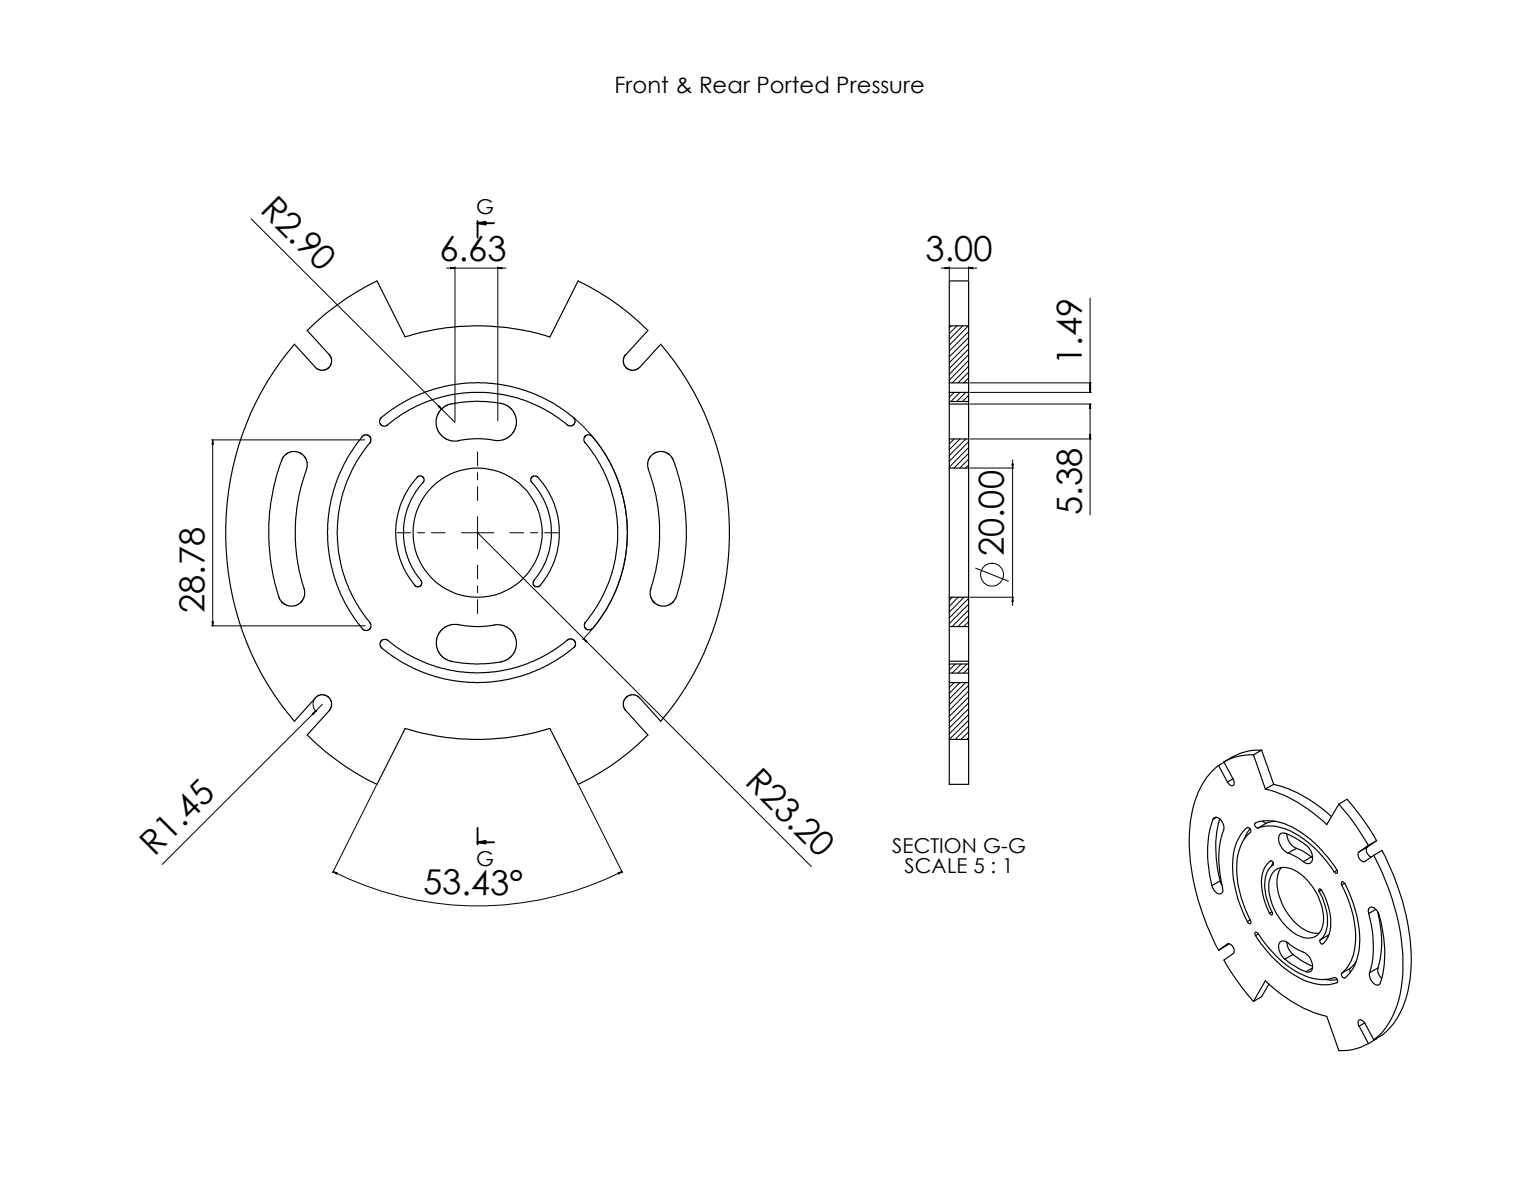
ISO-10303-21;
HEADER;
FILE_DESCRIPTION (('STEP AP214'),
    '1' );
FILE_NAME ('Front & Rear Ported Pressure.step',
    '2026-10-18T20:16:25',
    ( '' ),
    ( '' ),
    'SwSTEP 2.0',
    'SolidWorks 2025',
    '' );
FILE_SCHEMA (( 'AUTOMOTIVE_DESIGN' ));
ENDSEC;

DATA;
#15=ORIENTED_EDGE ( 'NONE', *, *, #5581, .T. ) ;
#25=AXIS2_PLACEMENT_3D ( 'NONE', #902, #17278, #15225 ) ;
#26=CARTESIAN_POINT ( 'NONE',  ( 30.75232512042845556, -9.966982604840845639, 1.500000000000000000 ) ) ;
#30=EDGE_CURVE ( 'NONE', #13253, #5262, #636, .T. ) ;
#59=ORIENTED_EDGE ( 'NONE', *, *, #6132, .F. ) ;
#63=EDGE_CURVE ( 'NONE', #25705, #14162, #9332, .T. ) ;
#81=CARTESIAN_POINT ( 'NONE',  ( -1.073881485057447405, -0.9711784013058452070, 1.500000000000000000 ) ) ;
#121=VECTOR ( 'NONE', #17231, 1000.000000000000000 ) ;
#142=AXIS2_PLACEMENT_3D ( 'NONE', #29835, #3468, #10482 ) ;
#156=DIRECTION ( 'NONE',  ( -0.000000000000000000, 0.000000000000000000, 1.000000000000000000 ) ) ;
#172=ORIENTED_EDGE ( 'NONE', *, *, #2713, .T. ) ;
#180=DIRECTION ( 'NONE',  ( 1.000000000000000000, 0.000000000000000000, 0.000000000000000000 ) ) ;
#190=DIRECTION ( 'NONE',  ( -0.6707505147970024284, 0.7416830501633134842, 0.000000000000000000 ) ) ;
#192=EDGE_CURVE ( 'NONE', #26671, #20986, #30262, .T. ) ;
#204=ORIENTED_EDGE ( 'NONE', *, *, #13604, .T. ) ;
#206=CIRCLE ( 'NONE', #4196, 0.7441270634457181066 ) ;
#213=CARTESIAN_POINT ( 'NONE',  ( -19.54426622602688113, -37.07991288358296345, -1.499999999999999778 ) ) ;
#244=CIRCLE ( 'NONE', #26653, 0.7441270634457198829 ) ;
#248=ORIENTED_EDGE ( 'NONE', *, *, #13418, .T. ) ;
#251=EDGE_CURVE ( 'NONE', #24781, #12321, #29562, .T. ) ;
#252=LINE ( 'NONE', #7437, #4085 ) ;
#265=EDGE_CURVE ( 'NONE', #30031, #12516, #9139, .T. ) ;
#274=DIRECTION ( 'NONE',  ( -0.000000000000000000, 0.000000000000000000, 1.000000000000000000 ) ) ;
#282=DIRECTION ( 'NONE',  ( -0.000000000000000000, -0.000000000000000000, -1.000000000000000000 ) ) ;
#288=AXIS2_PLACEMENT_3D ( 'NONE', #22323, #7993, #29353 ) ;
#292=ORIENTED_EDGE ( 'NONE', *, *, #27712, .F. ) ;
#317=AXIS2_PLACEMENT_3D ( 'NONE', #8530, #7913, #10548 ) ;
#320=DIRECTION ( 'NONE',  ( -1.000000000000000000, 0.000000000000000000, 0.000000000000000000 ) ) ;
#322=CYLINDRICAL_SURFACE ( 'NONE', #25724, 20.32284676574538906 ) ;
#374=CIRCLE ( 'NONE', #21296, 0.7441270634457181066 ) ;
#388=FACE_OUTER_BOUND ( 'NONE', #26241, .T. ) ;
#408=DIRECTION ( 'NONE',  ( -1.000000000000000000, 0.000000000000000000, 0.000000000000000000 ) ) ;
#409=ORIENTED_EDGE ( 'NONE', *, *, #20131, .F. ) ;
#423=AXIS2_PLACEMENT_3D ( 'NONE', #5251, #14749, #10546 ) ;
#429=EDGE_CURVE ( 'NONE', #25490, #7103, #10636, .T. ) ;
#442=ORIENTED_EDGE ( 'NONE', *, *, #12082, .T. ) ;
#450=EDGE_CURVE ( 'NONE', #9427, #25685, #22270, .T. ) ;
#468=CYLINDRICAL_SURFACE ( 'NONE', #18787, 2.898871837527149165 ) ;
#479=VERTEX_POINT ( 'NONE', #10583 ) ;
#481=CYLINDRICAL_SURFACE ( 'NONE', #1478, 0.6002263538043648428 ) ;
#486=ORIENTED_EDGE ( 'NONE', *, *, #11751, .F. ) ;
#491=LINE ( 'NONE', #29032, #2354 ) ;
#494=FACE_OUTER_BOUND ( 'NONE', #15914, .T. ) ;
#512=ORIENTED_EDGE ( 'NONE', *, *, #14149, .F. ) ;
#514=CARTESIAN_POINT ( 'NONE',  ( 9.216505592218814158, -7.781333699927420966, -1.500000000000000000 ) ) ;
#517=ORIENTED_EDGE ( 'NONE', *, *, #25356, .F. ) ;
#518=FACE_OUTER_BOUND ( 'NONE', #7310, .T. ) ;
#558=LINE ( 'NONE', #12121, #27803 ) ;
#568=LINE ( 'NONE', #26949, #28027 ) ;
#570=ORIENTED_EDGE ( 'NONE', *, *, #6962, .T. ) ;
#574=ADVANCED_BREP_SHAPE_REPRESENTATION ( '', ( #2768, #7396 ), #910 ) ;
#584=VERTEX_POINT ( 'NONE', #5059 ) ;
#597=ADVANCED_FACE ( 'NONE', ( #17058 ), #18881, .F. ) ;
#613=CARTESIAN_POINT ( 'NONE',  ( -4.100931858250860707, -19.90478481566557534, 1.500000000000000000 ) ) ;
#629=ORIENTED_EDGE ( 'NONE', *, *, #8754, .F. ) ;
#636=LINE ( 'NONE', #3142, #22778 ) ;
#652=EDGE_CURVE ( 'NONE', #15421, #2309, #4171, .T. ) ;
#663=CARTESIAN_POINT ( 'NONE',  ( -43.34097750826428097, -11.89502811014147987, -1.500000000000000444 ) ) ;
#666=CARTESIAN_POINT ( 'NONE',  ( -17.26937953831790651, 14.36006998371489551, -1.500000000000000000 ) ) ;
#686=FACE_OUTER_BOUND ( 'NONE', #13708, .T. ) ;
#701=CARTESIAN_POINT ( 'NONE',  ( -1.073881485057738949, 0.9711784013061123266, -1.500000000000000000 ) ) ;
#703=CARTESIAN_POINT ( 'NONE',  ( 26.36764545593177544, -31.31467416275353344, -1.500000000000000000 ) ) ;
#706=CARTESIAN_POINT ( 'NONE',  ( 24.03057240117691862, -26.57182937991349903, 1.500000000000000000 ) ) ;
#708=DIRECTION ( 'NONE',  ( 1.000000000000000000, 0.000000000000000000, 0.000000000000000000 ) ) ;
#717=DIRECTION ( 'NONE',  ( -0.000000000000000000, -0.000000000000000000, -1.000000000000000000 ) ) ;
#722=EDGE_LOOP ( 'NONE', ( #5355, #17765, #14254, #19084 ) ) ;
#733=( BOUNDED_CURVE ( )  B_SPLINE_CURVE ( 3, ( #29605, #26969, #8239, #8560 ),
 .UNSPECIFIED., .F., .T. ) 
 B_SPLINE_CURVE_WITH_KNOTS ( ( 4, 4 ),
 ( 3.955359442064654285, 5.469418518704724619 ),
 .UNSPECIFIED. ) 
 CURVE ( )  GEOMETRIC_REPRESENTATION_ITEM ( )  RATIONAL_B_SPLINE_CURVE ( ( 1.000000000000000000, 0.8179194830933629312, 0.8179194830933629312, 1.000000000000000000 ) ) 
 REPRESENTATION_ITEM ( '' )  );
#734=ORIENTED_EDGE ( 'NONE', *, *, #10715, .F. ) ;
#751=ADVANCED_FACE ( 'NONE', ( #22199 ), #1146, .F. ) ;
#763=ORIENTED_EDGE ( 'NONE', *, *, #27893, .T. ) ;
#775=CARTESIAN_POINT ( 'NONE',  ( 13.93942108199810193, -16.65122935894600076, 1.500000000000000000 ) ) ;
#791=ADVANCED_FACE ( 'NONE', ( #25481 ), #27968, .F. ) ;
#793=CIRCLE ( 'NONE', #3294, 2.061368542273053883 ) ;
#800=FACE_OUTER_BOUND ( 'NONE', #27813, .T. ) ;
#801=CARTESIAN_POINT ( 'NONE',  ( -4.163336342344337027E-14, -1.387778780781445676E-14, 1.500000000000000000 ) ) ;
#821=CARTESIAN_POINT ( 'NONE',  ( 0.000000000000000000, 0.000000000000000000, -1.500000000000000000 ) ) ;
#848=ORIENTED_EDGE ( 'NONE', *, *, #26955, .T. ) ;
#855=CIRCLE ( 'NONE', #18782, 1.447898107987198646 ) ;
#864=DIRECTION ( 'NONE',  ( -1.000000000000000000, 0.000000000000000000, 0.000000000000000000 ) ) ;
#871=AXIS2_PLACEMENT_3D ( 'NONE', #23570, #30756, #18919 ) ;
#876=CARTESIAN_POINT ( 'NONE',  ( 8.419710366748642372, 7.777014463793876509, 1.500000000000000000 ) ) ;
#889=VECTOR ( 'NONE', #15046, 1000.000000000000000 ) ;
#902=CARTESIAN_POINT ( 'NONE',  ( -4.163336342344337027E-14, -1.387778780781445676E-14, 1.500000000000000000 ) ) ;
#907=EDGE_CURVE ( 'NONE', #20436, #24781, #5018, .T. ) ;
#910=( GEOMETRIC_REPRESENTATION_CONTEXT ( 3 ) GLOBAL_UNCERTAINTY_ASSIGNED_CONTEXT ( ( #13624 ) ) GLOBAL_UNIT_ASSIGNED_CONTEXT ( ( #14769, #3081, #22254 ) ) REPRESENTATION_CONTEXT ( 'NONE', 'WORKASPACE' ) );
#927=ORIENTED_EDGE ( 'NONE', *, *, #27710, .F. ) ;
#953=EDGE_CURVE ( 'NONE', #29550, #14341, #3391, .T. ) ;
#955=CARTESIAN_POINT ( 'NONE',  ( -4.163336342344337027E-14, -1.387778780781445676E-14, -1.500000000000000000 ) ) ;
#958=CARTESIAN_POINT ( 'NONE',  ( -15.57266529552203416, -38.96488032230103471, 1.500000000000000000 ) ) ;
#973=CARTESIAN_POINT ( 'NONE',  ( -17.26937953831790651, 14.36006998371489551, 1.500000000000000000 ) ) ;
#986=CARTESIAN_POINT ( 'NONE',  ( -11.46182693247433804, -1.387778780781445676E-14, 1.500000000000000000 ) ) ;
#993=AXIS2_PLACEMENT_3D ( 'NONE', #30844, #28672, #23658 ) ;
#994=CARTESIAN_POINT ( 'NONE',  ( -23.17581250239728519, -34.50630206824673252, 1.499999999999999778 ) ) ;
#1017=AXIS2_PLACEMENT_3D ( 'NONE', #1740, #20609, #28248 ) ;
#1028=CYLINDRICAL_SURFACE ( 'NONE', #9384, 0.7441270634457198829 ) ;
#1036=EDGE_CURVE ( 'NONE', #3590, #15421, #14834, .T. ) ;
#1037=DIRECTION ( 'NONE',  ( -1.000000000000000000, 0.000000000000000000, 0.000000000000000000 ) ) ;
#1041=CARTESIAN_POINT ( 'NONE',  ( -43.34097750826428097, -11.89502811014148342, -1.500000000000000444 ) ) ;
#1046=DIRECTION ( 'NONE',  ( -0.000000000000000000, -0.000000000000000000, -1.000000000000000000 ) ) ;
#1049=ORIENTED_EDGE ( 'NONE', *, *, #3733, .T. ) ;
#1059=ORIENTED_EDGE ( 'NONE', *, *, #26955, .F. ) ;
#1073=CARTESIAN_POINT ( 'NONE',  ( -28.79137815760242702, -9.331429872129930914, 1.500000000000000000 ) ) ;
#1076=FACE_BOUND ( 'NONE', #3866, .T. ) ;
#1078=CARTESIAN_POINT ( 'NONE',  ( 15.57266529552203416, -38.96488032230103471, -1.500000000000000000 ) ) ;
#1105=VERTEX_POINT ( 'NONE', #15603 ) ;
#1106=DIRECTION ( 'NONE',  ( -1.000000000000000000, 0.000000000000000000, 0.000000000000000000 ) ) ;
#1108=DIRECTION ( 'NONE',  ( 1.000000000000000000, 0.000000000000000000, 0.000000000000000000 ) ) ;
#1113=AXIS2_PLACEMENT_3D ( 'NONE', #20021, #3967, #25158 ) ;
#1122=DIRECTION ( 'NONE',  ( 1.000000000000000000, 0.000000000000000000, 0.000000000000000000 ) ) ;
#1123=CARTESIAN_POINT ( 'NONE',  ( 24.03057240117691862, -26.57182937991349903, -1.500000000000000000 ) ) ;
#1135=VECTOR ( 'NONE', #24120, 1000.000000000000000 ) ;
#1138=CARTESIAN_POINT ( 'NONE',  ( -24.03057240117691862, -26.57182937991349903, 1.500000000000000000 ) ) ;
#1146=CYLINDRICAL_SURFACE ( 'NONE', #13138, 0.7441270634457181066 ) ;
#1158=ORIENTED_EDGE ( 'NONE', *, *, #15067, .F. ) ;
#1167=ORIENTED_EDGE ( 'NONE', *, *, #6161, .F. ) ;
#1172=EDGE_CURVE ( 'NONE', #27927, #23361, #4939, .T. ) ;
#1176=AXIS2_PLACEMENT_3D ( 'NONE', #4448, #24929, #1953 ) ;
#1177=ADVANCED_FACE ( 'NONE', ( #4517, #28690, #28535, #7328, #20890, #16837, #14027, #23530, #16679, #2176, #11399, #13884 ), #7011, .F. ) ;
#1185=LINE ( 'NONE', #5548, #28491 ) ;
#1202=FACE_OUTER_BOUND ( 'NONE', #13290, .T. ) ;
#1205=ORIENTED_EDGE ( 'NONE', *, *, #1997, .F. ) ;
#1212=DIRECTION ( 'NONE',  ( 1.000000000000000000, 0.000000000000000000, 0.000000000000000000 ) ) ;
#1236=FACE_OUTER_BOUND ( 'NONE', #7384, .T. ) ;
#1264=EDGE_CURVE ( 'NONE', #6747, #8400, #30302, .T. ) ;
#1265=LINE ( 'NONE', #18424, #21036 ) ;
#1272=DIRECTION ( 'NONE',  ( -0.000000000000000000, 0.000000000000000000, 1.000000000000000000 ) ) ;
#1275=CARTESIAN_POINT ( 'NONE',  ( -4.163336342344337027E-14, -1.387778780781445676E-14, 1.500000000000000000 ) ) ;
#1276=ORIENTED_EDGE ( 'NONE', *, *, #27924, .F. ) ;
#1277=ORIENTED_EDGE ( 'NONE', *, *, #5949, .F. ) ;
#1284=DIRECTION ( 'NONE',  ( -1.000000000000000000, 0.000000000000000000, 0.000000000000000000 ) ) ;
#1304=ORIENTED_EDGE ( 'NONE', *, *, #26374, .T. ) ;
#1329=DIRECTION ( 'NONE',  ( -1.000000000000000000, 0.000000000000000000, 0.000000000000000000 ) ) ;
#1341=CARTESIAN_POINT ( 'NONE',  ( -22.95669091611927826, -27.54300778121952220, 1.500000000000000000 ) ) ;
#1346=AXIS2_PLACEMENT_3D ( 'NONE', #18219, #6660, #16178 ) ;
#1352=VERTEX_POINT ( 'NONE', #5606 ) ;
#1358=DIRECTION ( 'NONE',  ( 1.000000000000000000, 0.000000000000000000, 0.000000000000000000 ) ) ;
#1360=ORIENTED_EDGE ( 'NONE', *, *, #7124, .F. ) ;
#1383=ADVANCED_FACE ( 'NONE', ( #20409, #22433, #24933, #13410, #30077, #1076, #24770, #15720, #11202, #3569, #10909, #15409 ), #29618, .T. ) ;
#1394=AXIS2_PLACEMENT_3D ( 'NONE', #19673, #26872, #10321 ) ;
#1397=CARTESIAN_POINT ( 'NONE',  ( 8.860628911697515875, 8.184276679720483116, 1.500000000000000000 ) ) ;
#1411=ORIENTED_EDGE ( 'NONE', *, *, #14365, .T. ) ;
#1416=LINE ( 'NONE', #3591, #23261 ) ;
#1427=CYLINDRICAL_SURFACE ( 'NONE', #14286, 0.7441270634457319844 ) ;
#1428=DIRECTION ( 'NONE',  ( -0.000000000000000000, -0.000000000000000000, -1.000000000000000000 ) ) ;
#1443=( LENGTH_UNIT ( ) NAMED_UNIT ( * ) SI_UNIT ( .MILLI., .METRE. ) );
#1449=ADVANCED_FACE ( 'NONE', ( #1236 ), #15568, .F. ) ;
#1460=CIRCLE ( 'NONE', #27926, 0.7441270634456903510 ) ;
#1462=ORIENTED_EDGE ( 'NONE', *, *, #19357, .F. ) ;
#1469=DIRECTION ( 'NONE',  ( -1.000000000000000000, 0.000000000000000000, 0.000000000000000000 ) ) ;
#1473=CIRCLE ( 'NONE', #23359, 2.061368542273053883 ) ;
#1478=AXIS2_PLACEMENT_3D ( 'NONE', #12501, #7807, #4847 ) ;
#1490=LINE ( 'NONE', #21948, #12448 ) ;
#1499=LINE ( 'NONE', #27688, #26304 ) ;
#1505=LINE ( 'NONE', #11014, #27746 ) ;
#1510=CARTESIAN_POINT ( 'NONE',  ( -16.69721919944057831, 13.88429941593312122, 1.500000000000000000 ) ) ;
#1513=VERTEX_POINT ( 'NONE', #16184 ) ;
#1514=ORIENTED_EDGE ( 'NONE', *, *, #15762, .F. ) ;
#1519=DIRECTION ( 'NONE',  ( -0.000000000000000000, 0.000000000000000000, 1.000000000000000000 ) ) ;
#1523=EDGE_LOOP ( 'NONE', ( #7018, #9466, #4233, #11567 ) ) ;
#1537=CARTESIAN_POINT ( 'NONE',  ( -11.21147646446735102, 30.29926891764210595, 1.500000000000000000 ) ) ;
#1542=DIRECTION ( 'NONE',  ( -0.000000000000000000, -0.000000000000000000, -1.000000000000000000 ) ) ;
#1571=ORIENTED_EDGE ( 'NONE', *, *, #2711, .T. ) ;
#1582=ORIENTED_EDGE ( 'NONE', *, *, #3226, .T. ) ;
#1596=DIRECTION ( 'NONE',  ( -0.000000000000000000, 0.000000000000000000, 1.000000000000000000 ) ) ;
#1611=EDGE_LOOP ( 'NONE', ( #27625, #4985, #27472, #29846 ) ) ;
#1625=DIRECTION ( 'NONE',  ( 1.000000000000000000, 0.000000000000000000, 0.000000000000000000 ) ) ;
#1632=DIRECTION ( 'NONE',  ( 1.000000000000000000, 0.000000000000000000, 0.000000000000000000 ) ) ;
#1633=VECTOR ( 'NONE', #3197, 1000.000000000000000 ) ;
#1651=DIRECTION ( 'NONE',  ( -0.000000000000000000, -0.000000000000000000, -1.000000000000000000 ) ) ;
#1675=FACE_OUTER_BOUND ( 'NONE', #11524, .T. ) ;
#1682=CARTESIAN_POINT ( 'NONE',  ( 17.79239818699415920, 14.89473990422378158, 1.500000000000000000 ) ) ;
#1707=CARTESIAN_POINT ( 'NONE',  ( -4.163336342344337027E-14, -1.387778780781445676E-14, -1.500000000000000000 ) ) ;
#1719=ORIENTED_EDGE ( 'NONE', *, *, #13952, .T. ) ;
#1725=VERTEX_POINT ( 'NONE', #12127 ) ;
#1727=CIRCLE ( 'NONE', #29633, 23.20393738267273420 ) ;
#1740=CARTESIAN_POINT ( 'NONE',  ( -4.163336342344337027E-14, 1.387778780781445676E-14, -1.500000000000000000 ) ) ;
#1743=ORIENTED_EDGE ( 'NONE', *, *, #12996, .F. ) ;
#1761=ADVANCED_FACE ( 'NONE', ( #19447 ), #14758, .F. ) ;
#1782=DIRECTION ( 'NONE',  ( -0.000000000000000000, -0.000000000000000000, -1.000000000000000000 ) ) ;
#1788=CARTESIAN_POINT ( 'NONE',  ( 17.84153987719590972, -14.83584055149750114, 1.500000000000000000 ) ) ;
#1800=CARTESIAN_POINT ( 'NONE',  ( 3.637110358602582583, 19.99473753024312117, 1.500000000000000000 ) ) ;
#1809=AXIS2_PLACEMENT_3D ( 'NONE', #13199, #12740, #10549 ) ;
#1821=CIRCLE ( 'NONE', #9786, 0.7441270634457337607 ) ;
#1831=CARTESIAN_POINT ( 'NONE',  ( 11.21147646446735102, 30.29926891764210595, -1.500000000000000000 ) ) ;
#1833=ORIENTED_EDGE ( 'NONE', *, *, #13418, .F. ) ;
#1834=AXIS2_PLACEMENT_3D ( 'NONE', #801, #3775, #24978 ) ;
#1851=CARTESIAN_POINT ( 'NONE',  ( -25.10445388623454477, 25.60065097860747585, -1.500000000000000000 ) ) ;
#1854=CARTESIAN_POINT ( 'NONE',  ( -23.20393738267338790, 0.000000000000000000, 1.500000000000000000 ) ) ;
#1856=ORIENTED_EDGE ( 'NONE', *, *, #17785, .F. ) ;
#1862=VECTOR ( 'NONE', #12585, 1000.000000000000000 ) ;
#1871=AXIS2_PLACEMENT_3D ( 'NONE', #12190, #16553, #28887 ) ;
#1876=ORIENTED_EDGE ( 'NONE', *, *, #23476, .F. ) ;
#1879=CIRCLE ( 'NONE', #15838, 1.447898107987198646 ) ;
#1884=VECTOR ( 'NONE', #29889, 1000.000000000000000 ) ;
#1914=CARTESIAN_POINT ( 'NONE',  ( -28.79137815760242702, -9.331429872129930914, 1.500000000000000000 ) ) ;
#1917=CARTESIAN_POINT ( 'NONE',  ( -25.10445388623454477, -25.60065097860747585, 1.500000000000000000 ) ) ;
#1921=AXIS2_PLACEMENT_3D ( 'NONE', #25373, #30355, #8997 ) ;
#1938=VECTOR ( 'NONE', #25198, 1000.000000000000000 ) ;
#1945=PLANE ( 'NONE',  #16481 ) ;
#1946=DIRECTION ( 'NONE',  ( 1.000000000000000000, 0.000000000000000000, 0.000000000000000000 ) ) ;
#1951=DIRECTION ( 'NONE',  ( 1.000000000000000000, 0.000000000000000000, 0.000000000000000000 ) ) ;
#1953=DIRECTION ( 'NONE',  ( 1.000000000000000000, -5.780230957810361426E-15, 0.000000000000000000 ) ) ;
#1997=EDGE_CURVE ( 'NONE', #27352, #27365, #19892, .T. ) ;
#2002=CARTESIAN_POINT ( 'NONE',  ( -13.88429941593315853, -16.69721919944146649, 1.500000000000000000 ) ) ;
#2003=ORIENTED_EDGE ( 'NONE', *, *, #16264, .T. ) ;
#2015=DIRECTION ( 'NONE',  ( -0.000000000000000000, -0.000000000000000000, -1.000000000000000000 ) ) ;
#2017=ORIENTED_EDGE ( 'NONE', *, *, #10988, .T. ) ;
#2042=ORIENTED_EDGE ( 'NONE', *, *, #21748, .F. ) ;
#2079=CARTESIAN_POINT ( 'NONE',  ( 28.79137815760242702, -9.331429872129930914, -1.500000000000000000 ) ) ;
#2090=DIRECTION ( 'NONE',  ( 1.000000000000000000, 0.000000000000000000, 0.000000000000000000 ) ) ;
#2108=CARTESIAN_POINT ( 'NONE',  ( -10.00000000000004263, 1.387778780781445676E-14, 1.500000000000000000 ) ) ;
#2110=EDGE_CURVE ( 'NONE', #16733, #28141, #22382, .T. ) ;
#2111=DIRECTION ( 'NONE',  ( 1.000000000000000000, 0.000000000000000000, 0.000000000000000000 ) ) ;
#2117=EDGE_CURVE ( 'NONE', #28435, #9405, #12931, .T. ) ;
#2125=VECTOR ( 'NONE', #190, 1000.000000000000000 ) ;
#2153=CIRCLE ( 'NONE', #29051, 37.60050224823048381 ) ;
#2171=VECTOR ( 'NONE', #29665, 1000.000000000000000 ) ;
#2176=FACE_BOUND ( 'NONE', #19630, .T. ) ;
#2206=CARTESIAN_POINT ( 'NONE',  ( 0.000000000000000000, 0.000000000000000000, 1.500000000000000000 ) ) ;
#2234=DIRECTION ( 'NONE',  ( 1.000000000000000000, 0.000000000000000000, 0.000000000000000000 ) ) ;
#2235=EDGE_CURVE ( 'NONE', #24520, #11332, #7958, .T. ) ;
#2255=ORIENTED_EDGE ( 'NONE', *, *, #24890, .F. ) ;
#2278=DIRECTION ( 'NONE',  ( -0.000000000000000000, -0.000000000000000000, -1.000000000000000000 ) ) ;
#2291=CARTESIAN_POINT ( 'NONE',  ( -22.95669091611927826, 27.54300778121952220, 1.500000000000000000 ) ) ;
#2309=VERTEX_POINT ( 'NONE', #18964 ) ;
#2354=VECTOR ( 'NONE', #3453, 1000.000000000000000 ) ;
#2370=CARTESIAN_POINT ( 'NONE',  ( 15.57266529552203416, 38.96488032230103471, -1.500000000000000000 ) ) ;
#2377=DIRECTION ( 'NONE',  ( -0.000000000000000000, -0.000000000000000000, -1.000000000000000000 ) ) ;
#2385=DIRECTION ( 'NONE',  ( -0.000000000000000000, -0.000000000000000000, -1.000000000000000000 ) ) ;
#2412=CARTESIAN_POINT ( 'NONE',  ( 15.57266529552201995, -38.96488032230103471, -1.500000000000000000 ) ) ;
#2414=AXIS2_PLACEMENT_3D ( 'NONE', #24888, #24716, #22392 ) ;
#2422=CARTESIAN_POINT ( 'NONE',  ( 17.79239818699415920, 14.89473990422378158, -1.500000000000000000 ) ) ;
#2423=ADVANCED_FACE ( 'NONE', ( #686 ), #28623, .T. ) ;
#2436=VECTOR ( 'NONE', #10712, 1000.000000000000000 ) ;
#2441=AXIS2_PLACEMENT_3D ( 'NONE', #28161, #6956, #2111 ) ;
#2447=LINE ( 'NONE', #11967, #11055 ) ;
#2453=CARTESIAN_POINT ( 'NONE',  ( 8.616279238414451314, -7.781333699927420966, 1.500000000000000000 ) ) ;
#2456=DIRECTION ( 'NONE',  ( -0.8932538319083086487, -0.4495526574063634095, 0.000000000000000000 ) ) ;
#2467=CARTESIAN_POINT ( 'NONE',  ( -22.95669091611927826, 27.54300778121952220, -1.500000000000000000 ) ) ;
#2480=AXIS2_PLACEMENT_3D ( 'NONE', #23136, #11458, #20941 ) ;
#2515=EDGE_CURVE ( 'NONE', #24825, #14826, #23426, .T. ) ;
#2517=VERTEX_POINT ( 'NONE', #21699 ) ;
#2528=DIRECTION ( 'NONE',  ( -0.000000000000000000, -0.000000000000000000, -1.000000000000000000 ) ) ;
#2536=CARTESIAN_POINT ( 'NONE',  ( -3.221450758838616757, 1.621276839356792454, -1.500000000000000000 ) ) ;
#2551=VERTEX_POINT ( 'NONE', #11908 ) ;
#2554=EDGE_LOOP ( 'NONE', ( #25894, #27667, #22850, #11057, #23980, #17264 ) ) ;
#2567=CARTESIAN_POINT ( 'NONE',  ( -26.36764545593177544, -31.31467416275353344, -1.500000000000000000 ) ) ;
#2584=DIRECTION ( 'NONE',  ( -1.000000000000000000, 0.000000000000000000, 0.000000000000000000 ) ) ;
#2593=VECTOR ( 'NONE', #21769, 1000.000000000000000 ) ;
#2601=CARTESIAN_POINT ( 'NONE',  ( -1.073881485057887497, 0.9711784013062738641, 1.500000000000000000 ) ) ;
#2604=LINE ( 'NONE', #2761, #2830 ) ;
#2618=CARTESIAN_POINT ( 'NONE',  ( 17.22181377297005866, 14.41708049311048789, -1.500000000000000000 ) ) ;
#2655=VECTOR ( 'NONE', #25234, 1000.000000000000000 ) ;
#2656=DIRECTION ( 'NONE',  ( -1.000000000000000000, 0.000000000000000000, 0.000000000000000000 ) ) ;
#2668=ORIENTED_EDGE ( 'NONE', *, *, #18963, .F. ) ;
#2672=ORIENTED_EDGE ( 'NONE', *, *, #5239, .T. ) ;
#2697=DIRECTION ( 'NONE',  ( -0.000000000000000000, 0.000000000000000000, 1.000000000000000000 ) ) ;
#2704=ORIENTED_EDGE ( 'NONE', *, *, #23249, .T. ) ;
#2710=CIRCLE ( 'NONE', #10186, 2.061368542273053883 ) ;
#2711=EDGE_CURVE ( 'NONE', #23725, #7065, #19746, .T. ) ;
#2713=EDGE_CURVE ( 'NONE', #26988, #12630, #8473, .T. ) ;
#2724=EDGE_CURVE ( 'NONE', #2309, #20990, #15232, .T. ) ;
#2755=LINE ( 'NONE', #12267, #2593 ) ;
#2761=CARTESIAN_POINT ( 'NONE',  ( 26.31795596221988376, 10.51822134874671022, 1.500000000000000000 ) ) ;
#2768=MANIFOLD_SOLID_BREP ( 'Boss-Extrude1', #19793 ) ;
#2773=CARTESIAN_POINT ( 'NONE',  ( -4.163336342344337027E-14, -1.387778780781445676E-14, 1.500000000000000000 ) ) ;
#2791=CARTESIAN_POINT ( 'NONE',  ( -19.54426622602688468, 37.07991288358297055, 1.499999999999999778 ) ) ;
#2795=DIRECTION ( 'NONE',  ( 1.000000000000000000, 0.000000000000000000, 0.000000000000000000 ) ) ;
#2826=FACE_OUTER_BOUND ( 'NONE', #17698, .T. ) ;
#2830=VECTOR ( 'NONE', #4942, 1000.000000000000000 ) ;
#2841=AXIS2_PLACEMENT_3D ( 'NONE', #29655, #26695, #8292 ) ;
#2843=CARTESIAN_POINT ( 'NONE',  ( -1.073881485057738949, -0.9711784013061123266, -1.500000000000000000 ) ) ;
#2875=VECTOR ( 'NONE', #15795, 1000.000000000000000 ) ;
#2886=CARTESIAN_POINT ( 'NONE',  ( 15.57266529552203416, 38.96488032230103471, 1.500000000000000000 ) ) ;
#2892=CARTESIAN_POINT ( 'NONE',  ( -11.46182693247433804, -1.387778780781445676E-14, 1.500000000000000000 ) ) ;
#2913=DIRECTION ( 'NONE',  ( -0.000000000000000000, -0.000000000000000000, -1.000000000000000000 ) ) ;
#2924=ADVANCED_FACE ( 'NONE', ( #11512 ), #27736, .T. ) ;
#2929=CARTESIAN_POINT ( 'NONE',  ( -28.37932450449293853, 10.51822134874671022, 1.500000000000000000 ) ) ;
#2930=CARTESIAN_POINT ( 'NONE',  ( -10.00000000000004263, 1.387778780781445676E-14, 1.500000000000000000 ) ) ;
#2940=AXIS2_PLACEMENT_3D ( 'NONE', #21597, #18970, #2584 ) ;
#2943=ADVANCED_FACE ( 'NONE', ( #16027 ), #30379, .F. ) ;
#2949=DIRECTION ( 'NONE',  ( -0.000000000000000000, -0.000000000000000000, -1.000000000000000000 ) ) ;
#2970=DIRECTION ( 'NONE',  ( -1.000000000000000000, 0.000000000000000000, 0.000000000000000000 ) ) ;
#2980=ORIENTED_EDGE ( 'NONE', *, *, #15496, .T. ) ;
#2985=CIRCLE ( 'NONE', #17437, 2.061368542273053883 ) ;
#2993=CARTESIAN_POINT ( 'NONE',  ( 30.31220697679117038, 11.23460505553742550, 1.500000000000000000 ) ) ;
#2994=CARTESIAN_POINT ( 'NONE',  ( -19.54426622602688468, -37.07991288358296345, -1.499999999999999778 ) ) ;
#3010=VERTEX_POINT ( 'NONE', #5410 ) ;
#3026=DIRECTION ( 'NONE',  ( 1.000000000000000000, 0.000000000000000000, 0.000000000000000000 ) ) ;
#3040=ORIENTED_EDGE ( 'NONE', *, *, #25557, .F. ) ;
#3078=EDGE_CURVE ( 'NONE', #20938, #6747, #12437, .T. ) ;
#3081=( NAMED_UNIT ( * ) PLANE_ANGLE_UNIT ( ) SI_UNIT ( $, .RADIAN. ) );
#3087=ORIENTED_EDGE ( 'NONE', *, *, #30388, .T. ) ;
#3095=EDGE_CURVE ( 'NONE', #10630, #4361, #28500, .T. ) ;
#3100=EDGE_CURVE ( 'NONE', #14341, #26022, #2604, .T. ) ;
#3115=ORIENTED_EDGE ( 'NONE', *, *, #21996, .T. ) ;
#3139=CARTESIAN_POINT ( 'NONE',  ( -4.163336342344337027E-14, 1.387778780781445676E-14, 1.500000000000000000 ) ) ;
#3140=AXIS2_PLACEMENT_3D ( 'NONE', #24833, #1596, #8612 ) ;
#3142=CARTESIAN_POINT ( 'NONE',  ( -21.71568325578193637, 0.000000000000000000, 1.500000000000000000 ) ) ;
#3143=DIRECTION ( 'NONE',  ( -0.000000000000000000, -0.000000000000000000, -1.000000000000000000 ) ) ;
#3160=EDGE_CURVE ( 'NONE', #5226, #1513, #29453, .T. ) ;
#3169=VERTEX_POINT ( 'NONE', #8369 ) ;
#3178=CARTESIAN_POINT ( 'NONE',  ( -19.54426622602688113, -37.07991288358296345, 1.499999999999999778 ) ) ;
#3195=LINE ( 'NONE', #2892, #25607 ) ;
#3197=DIRECTION ( 'NONE',  ( -0.000000000000000000, -0.000000000000000000, -1.000000000000000000 ) ) ;
#3226=EDGE_CURVE ( 'NONE', #28141, #26677, #14733, .T. ) ;
#3229=ORIENTED_EDGE ( 'NONE', *, *, #29002, .F. ) ;
#3234=CARTESIAN_POINT ( 'NONE',  ( 13.88429941593329531, 16.69721919943964039, -1.500000000000000000 ) ) ;
#3242=EDGE_CURVE ( 'NONE', #14300, #23449, #28183, .T. ) ;
#3260=EDGE_CURVE ( 'NONE', #27498, #8808, #6482, .T. ) ;
#3265=DIRECTION ( 'NONE',  ( -0.000000000000000000, -0.000000000000000000, -1.000000000000000000 ) ) ;
#3294=AXIS2_PLACEMENT_3D ( 'NONE', #17421, #18036, #8372 ) ;
#3295=DIRECTION ( 'NONE',  ( 1.000000000000000000, 4.440892098500626162E-15, 0.000000000000000000 ) ) ;
#3303=CARTESIAN_POINT ( 'NONE',  ( -8.419710366748644148, 7.777014463793872956, 1.500000000000000000 ) ) ;
#3304=EDGE_CURVE ( 'NONE', #10421, #30261, #25815, .T. ) ;
#3308=ORIENTED_EDGE ( 'NONE', *, *, #6548, .T. ) ;
#3317=DIRECTION ( 'NONE',  ( -1.000000000000000000, 0.000000000000000000, 0.000000000000000000 ) ) ;
#3337=DIRECTION ( 'NONE',  ( -0.000000000000000000, -0.000000000000000000, -1.000000000000000000 ) ) ;
#3343=VERTEX_POINT ( 'NONE', #9438 ) ;
#3349=VERTEX_POINT ( 'NONE', #19556 ) ;
#3354=VERTEX_POINT ( 'NONE', #9891 ) ;
#3356=CARTESIAN_POINT ( 'NONE',  ( 23.17581250239727808, -34.50630206824672541, -1.499999999999999778 ) ) ;
#3359=CARTESIAN_POINT ( 'NONE',  ( -4.100931858250869588, 19.90478481566557178, 1.500000000000000000 ) ) ;
#3365=AXIS2_PLACEMENT_3D ( 'NONE', #15998, #25517, #3994 ) ;
#3369=CARTESIAN_POINT ( 'NONE',  ( 15.57266529552203416, 38.96488032230103471, -1.500000000000000000 ) ) ;
#3371=FACE_OUTER_BOUND ( 'NONE', #22200, .T. ) ;
#3382=DIRECTION ( 'NONE',  ( -0.000000000000000000, -0.000000000000000000, -1.000000000000000000 ) ) ;
#3386=DIRECTION ( 'NONE',  ( 1.000000000000000000, 0.000000000000000000, 0.000000000000000000 ) ) ;
#3391=CIRCLE ( 'NONE', #11875, 2.061368542273053883 ) ;
#3397=AXIS2_PLACEMENT_3D ( 'NONE', #19127, #28495, #28795 ) ;
#3424=CARTESIAN_POINT ( 'NONE',  ( 8.260402557893151254, 8.184276679720483116, 1.500000000000000000 ) ) ;
#3431=ORIENTED_EDGE ( 'NONE', *, *, #17583, .T. ) ;
#3437=ORIENTED_EDGE ( 'NONE', *, *, #3078, .F. ) ;
#3443=ORIENTED_EDGE ( 'NONE', *, *, #953, .F. ) ;
#3452=LINE ( 'NONE', #958, #4921 ) ;
#3453=DIRECTION ( 'NONE',  ( -0.000000000000000000, -0.000000000000000000, -1.000000000000000000 ) ) ;
#3461=DIRECTION ( 'NONE',  ( 0.000000000000000000, -0.000000000000000000, -1.000000000000000000 ) ) ;
#3465=EDGE_CURVE ( 'NONE', #8846, #28935, #25201, .T. ) ;
#3468=DIRECTION ( 'NONE',  ( -0.000000000000000000, 0.000000000000000000, 1.000000000000000000 ) ) ;
#3469=AXIS2_PLACEMENT_3D ( 'NONE', #3779, #22794, #16088 ) ;
#3474=ORIENTED_EDGE ( 'NONE', *, *, #4046, .T. ) ;
#3475=AXIS2_PLACEMENT_3D ( 'NONE', #20573, #2015, #30548 ) ;
#3480=ORIENTED_EDGE ( 'NONE', *, *, #26926, .T. ) ;
#3485=FACE_OUTER_BOUND ( 'NONE', #4334, .T. ) ;
#3490=EDGE_CURVE ( 'NONE', #12630, #30261, #7258, .T. ) ;
#3493=CARTESIAN_POINT ( 'NONE',  ( -26.36764545593177544, -31.31467416275353344, 1.500000000000000000 ) ) ;
#3523=ADVANCED_FACE ( 'NONE', ( #26824 ), #18689, .F. ) ;
#3531=CARTESIAN_POINT ( 'NONE',  ( -4.163336342344337027E-14, 1.387778780781445676E-14, 1.500000000000000000 ) ) ;
#3542=EDGE_LOOP ( 'NONE', ( #28191, #26156, #18227, #7416, #17416 ) ) ;
#3554=VECTOR ( 'NONE', #5605, 1000.000000000000000 ) ;
#3568=CARTESIAN_POINT ( 'NONE',  ( -15.57266529552203416, 38.96488032230103471, 1.500000000000000000 ) ) ;
#3569=FACE_BOUND ( 'NONE', #20676, .T. ) ;
#3576=VERTEX_POINT ( 'NONE', #13244 ) ;
#3588=CARTESIAN_POINT ( 'NONE',  ( 0.000000000000000000, 5.590849009245238754, -1.500000000000000000 ) ) ;
#3590=VERTEX_POINT ( 'NONE', #27740 ) ;
#3591=CARTESIAN_POINT ( 'NONE',  ( -1.073881485057447405, -0.9711784013058452070, -1.500000000000000000 ) ) ;
#3593=FACE_OUTER_BOUND ( 'NONE', #29538, .T. ) ;
#3607=DIRECTION ( 'NONE',  ( 1.000000000000000000, 0.000000000000000000, 0.000000000000000000 ) ) ;
#3617=LINE ( 'NONE', #3303, #2171 ) ;
#3628=AXIS2_PLACEMENT_3D ( 'NONE', #19070, #9558, #28590 ) ;
#3639=LINE ( 'NONE', #22647, #4104 ) ;
#3642=ADVANCED_FACE ( 'NONE', ( #10433 ), #22430, .F. ) ;
#3677=DIRECTION ( 'NONE',  ( -1.000000000000000000, 0.000000000000000000, 0.000000000000000000 ) ) ;
#3686=ADVANCED_FACE ( 'NONE', ( #30520 ), #18839, .F. ) ;
#3689=CARTESIAN_POINT ( 'NONE',  ( -43.34097750826428097, 11.89502811014148342, -1.500000000000000444 ) ) ;
#3718=ORIENTED_EDGE ( 'NONE', *, *, #21167, .F. ) ;
#3719=DIRECTION ( 'NONE',  ( -0.000000000000000000, -0.000000000000000000, -1.000000000000000000 ) ) ;
#3730=DIRECTION ( 'NONE',  ( -1.000000000000000000, 0.000000000000000000, 0.000000000000000000 ) ) ;
#3733=EDGE_CURVE ( 'NONE', #28942, #6434, #23641, .T. ) ;
#3741=ORIENTED_EDGE ( 'NONE', *, *, #5727, .F. ) ;
#3751=ORIENTED_EDGE ( 'NONE', *, *, #17241, .T. ) ;
#3756=DIRECTION ( 'NONE',  ( -1.000000000000000000, 0.000000000000000000, 0.000000000000000000 ) ) ;
#3758=ORIENTED_EDGE ( 'NONE', *, *, #25426, .T. ) ;
#3775=DIRECTION ( 'NONE',  ( -0.000000000000000000, 0.000000000000000000, 1.000000000000000000 ) ) ;
#3779=CARTESIAN_POINT ( 'NONE',  ( 17.22181377297005866, 14.41708049311048789, 1.500000000000000000 ) ) ;
#3788=CIRCLE ( 'NONE', #9765, 37.60050224823048381 ) ;
#3790=ORIENTED_EDGE ( 'NONE', *, *, #7461, .T. ) ;
#3794=DIRECTION ( 'NONE',  ( 1.000000000000000000, 0.000000000000000000, 0.000000000000000000 ) ) ;
#3799=EDGE_LOOP ( 'NONE', ( #20233, #10447, #19766, #14062 ) ) ;
#3820=EDGE_LOOP ( 'NONE', ( #8228, #19617, #18856, #20756, #29475, #27058 ) ) ;
#3830=ORIENTED_EDGE ( 'NONE', *, *, #9612, .F. ) ;
#3846=ORIENTED_EDGE ( 'NONE', *, *, #12257, .F. ) ;
#3847=VERTEX_POINT ( 'NONE', #9627 ) ;
#3866=EDGE_LOOP ( 'NONE', ( #512, #4687, #24905, #11331, #27886 ) ) ;
#3893=ORIENTED_EDGE ( 'NONE', *, *, #3260, .F. ) ;
#3907=ORIENTED_EDGE ( 'NONE', *, *, #7057, .F. ) ;
#3913=PRODUCT_DEFINITION_CONTEXT ( 'detailed design', #26935, 'design' ) ;
#3916=ORIENTED_EDGE ( 'NONE', *, *, #22807, .T. ) ;
#3923=VECTOR ( 'NONE', #6766, 1000.000000000000000 ) ;
#3947=CARTESIAN_POINT ( 'NONE',  ( -4.163336342344337027E-14, -1.387778780781445676E-14, 1.500000000000000000 ) ) ;
#3951=FACE_OUTER_BOUND ( 'NONE', #16122, .T. ) ;
#3954=( BOUNDED_SURFACE ( )  B_SPLINE_SURFACE ( 3, 1, ( 
 ( #26391, #12354 ),
 ( #19518, #12667 ),
 ( #5323, #2994 ),
 ( #15286, #12971 ) ),
 .UNSPECIFIED., .F., .F., .T. ) 
 B_SPLINE_SURFACE_WITH_KNOTS ( ( 4, 4 ),
 ( 2, 2 ),
 ( 0.000000000000000000, 1.000000000000000000 ),
 ( 0.000000000000000000, 1.000000000000000000 ),
 .UNSPECIFIED. ) 
 GEOMETRIC_REPRESENTATION_ITEM ( )  RATIONAL_B_SPLINE_SURFACE ( (
 ( 1.000000000000000000, 1.000000000000000000),
 ( 0.9908525036704132205, 0.9908525036704132205),
 ( 0.9908525036704132205, 0.9908525036704132205),
 ( 1.000000000000000000, 1.000000000000000000) ) ) 
 REPRESENTATION_ITEM ( '' )  SURFACE ( )  );
#3967=DIRECTION ( 'NONE',  ( -0.000000000000000000, 0.000000000000000000, 1.000000000000000000 ) ) ;
#3983=CARTESIAN_POINT ( 'NONE',  ( 0.000000000000000000, 0.000000000000000000, 1.500000000000000000 ) ) ;
#3989=VERTEX_POINT ( 'NONE', #19137 ) ;
#3992=CARTESIAN_POINT ( 'NONE',  ( 15.57266529552203416, -38.96488032230103471, 1.500000000000000000 ) ) ;
#3994=DIRECTION ( 'NONE',  ( 1.000000000000000000, 0.000000000000000000, 0.000000000000000000 ) ) ;
#4003=CARTESIAN_POINT ( 'NONE',  ( 28.34828976096172681, 29.18752572968383419, -1.500000000000000000 ) ) ;
#4019=EDGE_CURVE ( 'NONE', #6841, #26671, #13287, .T. ) ;
#4022=LINE ( 'NONE', #13844, #14811 ) ;
#4042=DIRECTION ( 'NONE',  ( -0.000000000000000000, -0.000000000000000000, -1.000000000000000000 ) ) ;
#4046=EDGE_CURVE ( 'NONE', #19640, #26022, #793, .T. ) ;
#4054=EDGE_CURVE ( 'NONE', #24825, #21731, #9306, .T. ) ;
#4062=VECTOR ( 'NONE', #15681, 1000.000000000000000 ) ;
#4073=FACE_OUTER_BOUND ( 'NONE', #22551, .T. ) ;
#4074=EDGE_CURVE ( 'NONE', #19699, #4573, #15229, .T. ) ;
#4075=VECTOR ( 'NONE', #16182, 1000.000000000000000 ) ;
#4085=VECTOR ( 'NONE', #30821, 1000.000000000000000 ) ;
#4098=CARTESIAN_POINT ( 'NONE',  ( 28.37932450449293853, 10.51822134874671022, 1.500000000000000000 ) ) ;
#4101=DIRECTION ( 'NONE',  ( -0.000000000000000000, 0.000000000000000000, 1.000000000000000000 ) ) ;
#4104=VECTOR ( 'NONE', #6592, 1000.000000000000114 ) ;
#4113=CARTESIAN_POINT ( 'NONE',  ( -23.17581250239728519, 34.50630206824672541, 1.499999999999999778 ) ) ;
#4120=AXIS2_PLACEMENT_3D ( 'NONE', #13060, #10867, #22550 ) ;
#4125=DIRECTION ( 'NONE',  ( 0.000000000000000000, -0.000000000000000000, -1.000000000000000000 ) ) ;
#4137=AXIS2_PLACEMENT_3D ( 'NONE', #973, #12834, #20459 ) ;
#4138=DIRECTION ( 'NONE',  ( -1.000000000000000000, 0.000000000000000000, 0.000000000000000000 ) ) ;
#4141=CARTESIAN_POINT ( 'NONE',  ( -3.515970705488605130, -17.06554576617236307, 1.500000000000000000 ) ) ;
#4147=ORIENTED_EDGE ( 'NONE', *, *, #4054, .F. ) ;
#4158=CIRCLE ( 'NONE', #13143, 23.20393738267338790 ) ;
#4171=CIRCLE ( 'NONE', #11154, 23.20393738267338790 ) ;
#4196=AXIS2_PLACEMENT_3D ( 'NONE', #2618, #274, #28200 ) ;
#4199=EDGE_LOOP ( 'NONE', ( #517, #16025, #16239, #292, #1167, #17865, #20571, #17192, #27539, #4262, #21843, #21431, #5471, #14410, #5926, #20078, #24138, #24209, #12133, #7149, #26635, #2017, #7569, #20691, #3431, #9511 ) ) ;
#4223=CARTESIAN_POINT ( 'NONE',  ( 9.216505592218814158, -7.781333699927420966, 1.500000000000000000 ) ) ;
#4228=DIRECTION ( 'NONE',  ( -1.000000000000000000, 0.000000000000000000, 0.000000000000000000 ) ) ;
#4232=FACE_OUTER_BOUND ( 'NONE', #30300, .T. ) ;
#4233=ORIENTED_EDGE ( 'NONE', *, *, #16442, .T. ) ;
#4240=CARTESIAN_POINT ( 'NONE',  ( -4.163336342344337027E-14, 1.387778780781445676E-14, 1.500000000000000000 ) ) ;
#4244=CARTESIAN_POINT ( 'NONE',  ( -3.515970705488605130, -17.06554576617236307, 1.500000000000000000 ) ) ;
#4246=EDGE_LOOP ( 'NONE', ( #3474, #28596, #25128, #21949, #3916, #27127 ) ) ;
#4262=ORIENTED_EDGE ( 'NONE', *, *, #9922, .T. ) ;
#4273=ADVANCED_FACE ( 'NONE', ( #29691 ), #5523, .F. ) ;
#4275=DIRECTION ( 'NONE',  ( 0.8932538319083086487, -0.4495526574063634095, 0.000000000000000000 ) ) ;
#4288=DIRECTION ( 'NONE',  ( 1.000000000000000000, 4.440892098500625373E-15, 0.000000000000000000 ) ) ;
#4294=CARTESIAN_POINT ( 'NONE',  ( -28.79137815760242702, -9.331429872129930914, -1.500000000000000000 ) ) ;
#4302=ORIENTED_EDGE ( 'NONE', *, *, #18529, .T. ) ;
#4313=DIRECTION ( 'NONE',  ( 1.000000000000000000, 0.000000000000000000, 0.000000000000000000 ) ) ;
#4323=AXIS2_PLACEMENT_3D ( 'NONE', #5483, #3143, #8135 ) ;
#4329=ORIENTED_EDGE ( 'NONE', *, *, #30067, .F. ) ;
#4334=EDGE_LOOP ( 'NONE', ( #11368, #25411, #409, #25739 ) ) ;
#4342=ORIENTED_EDGE ( 'NONE', *, *, #28074, .F. ) ;
#4348=EDGE_LOOP ( 'NONE', ( #8219, #11418, #25052, #23025 ) ) ;
#4360=CARTESIAN_POINT ( 'NONE',  ( -28.34828976096172681, -29.18752572968383419, 1.500000000000000000 ) ) ;
#4361=VERTEX_POINT ( 'NONE', #29864 ) ;
#4380=ORIENTED_EDGE ( 'NONE', *, *, #24844, .T. ) ;
#4388=VERTEX_POINT ( 'NONE', #5836 ) ;
#4393=ORIENTED_EDGE ( 'NONE', *, *, #7277, .T. ) ;
#4399=CYLINDRICAL_SURFACE ( 'NONE', #20325, 2.061368542273053883 ) ;
#4405=ORIENTED_EDGE ( 'NONE', *, *, #28416, .T. ) ;
#4411=DIRECTION ( 'NONE',  ( -0.000000000000000000, 0.000000000000000000, 1.000000000000000000 ) ) ;
#4416=AXIS2_PLACEMENT_3D ( 'NONE', #20527, #10562, #1358 ) ;
#4444=ADVANCED_FACE ( 'NONE', ( #21076 ), #28121, .F. ) ;
#4448=CARTESIAN_POINT ( 'NONE',  ( -9.216505592218814158, -7.781333699927420966, 1.500000000000000000 ) ) ;
#4465=CARTESIAN_POINT ( 'NONE',  ( 14.89473990422475680, -17.79239818699420539, 1.500000000000000000 ) ) ;
#4466=VERTEX_POINT ( 'NONE', #25634 ) ;
#4511=DIRECTION ( 'NONE',  ( 1.000000000000000000, 0.000000000000000000, 0.000000000000000000 ) ) ;
#4517=FACE_BOUND ( 'NONE', #19816, .T. ) ;
#4525=ORIENTED_EDGE ( 'NONE', *, *, #21854, .F. ) ;
#4533=ORIENTED_EDGE ( 'NONE', *, *, #15839, .T. ) ;
#4551=CARTESIAN_POINT ( 'NONE',  ( -10.00000000000004263, 1.387778780781445676E-14, -1.500000000000000000 ) ) ;
#4554=CIRCLE ( 'NONE', #28965, 11.46182693247435935 ) ;
#4573=VERTEX_POINT ( 'NONE', #16718 ) ;
#4581=VERTEX_POINT ( 'NONE', #17025 ) ;
#4592=CARTESIAN_POINT ( 'NONE',  ( 26.36764545593177544, -31.31467416275353344, 1.500000000000000000 ) ) ;
#4610=EDGE_CURVE ( 'NONE', #18893, #6285, #25275, .T. ) ;
#4611=CARTESIAN_POINT ( 'NONE',  ( -14.36006998371493637, -17.26937953831884442, 1.500000000000000000 ) ) ;
#4618=ORIENTED_EDGE ( 'NONE', *, *, #6709, .F. ) ;
#4625=EDGE_CURVE ( 'NONE', #21504, #5226, #7678, .T. ) ;
#4630=ORIENTED_EDGE ( 'NONE', *, *, #21768, .F. ) ;
#4670=CARTESIAN_POINT ( 'NONE',  ( -43.34097750826428097, -11.89502811014148342, 1.500000000000000444 ) ) ;
#4687=ORIENTED_EDGE ( 'NONE', *, *, #4074, .F. ) ;
#4699=CARTESIAN_POINT ( 'NONE',  ( -17.79239818699324616, -14.89473990422481187, 1.500000000000000000 ) ) ;
#4716=CARTESIAN_POINT ( 'NONE',  ( -15.10419704716067102, -17.26937953831884442, -1.500000000000000000 ) ) ;
#4746=FACE_OUTER_BOUND ( 'NONE', #22612, .T. ) ;
#4750=CARTESIAN_POINT ( 'NONE',  ( 1.073881485057758711, -0.9711784013061475207, -1.500000000000000000 ) ) ;
#4768=EDGE_CURVE ( 'NONE', #4932, #21725, #29265, .T. ) ;
#4774=EDGE_CURVE ( 'NONE', #26376, #14162, #5344, .T. ) ;
#4795=CIRCLE ( 'NONE', #17249, 2.061368542273053883 ) ;
#4801=ORIENTED_EDGE ( 'NONE', *, *, #17400, .T. ) ;
#4818=DIRECTION ( 'NONE',  ( -0.000000000000000000, 0.000000000000000000, 1.000000000000000000 ) ) ;
#4825=ORIENTED_EDGE ( 'NONE', *, *, #7691, .T. ) ;
#4832=VECTOR ( 'NONE', #17699, 1000.000000000000000 ) ;
#4836=ORIENTED_EDGE ( 'NONE', *, *, #12611, .T. ) ;
#4847=DIRECTION ( 'NONE',  ( -1.000000000000000000, 0.000000000000000000, 0.000000000000000000 ) ) ;
#4859=VECTOR ( 'NONE', #2278, 1000.000000000000000 ) ;
#4864=VECTOR ( 'NONE', #24722, 1000.000000000000000 ) ;
#4875=AXIS2_PLACEMENT_3D ( 'NONE', #10231, #7915, #18189 ) ;
#4877=DIRECTION ( 'NONE',  ( -1.000000000000000000, 0.000000000000000000, 0.000000000000000000 ) ) ;
#4880=ORIENTED_EDGE ( 'NONE', *, *, #19250, .F. ) ;
#4909=DIRECTION ( 'NONE',  ( 0.8932538319083086487, 0.4495526574063634095, -0.000000000000000000 ) ) ;
#4921=VECTOR ( 'NONE', #29031, 1000.000000000000000 ) ;
#4932=VERTEX_POINT ( 'NONE', #26043 ) ;
#4939=( BOUNDED_CURVE ( )  B_SPLINE_CURVE ( 3, ( #26353, #26038, #4670, #4360 ),
 .UNSPECIFIED., .F., .T. ) 
 B_SPLINE_CURVE_WITH_KNOTS ( ( 4, 4 ),
 ( 0.8137667884748612801, 2.327825865114931947 ),
 .UNSPECIFIED. ) 
 CURVE ( )  GEOMETRIC_REPRESENTATION_ITEM ( )  RATIONAL_B_SPLINE_CURVE ( ( 1.000000000000000000, 0.8179194830933627092, 0.8179194830933627092, 1.000000000000000000 ) ) 
 REPRESENTATION_ITEM ( '' )  );
#4941=DIRECTION ( 'NONE',  ( -0.000000000000000000, 0.000000000000000000, 1.000000000000000000 ) ) ;
#4942=DIRECTION ( 'NONE',  ( -0.000000000000000000, -0.000000000000000000, -1.000000000000000000 ) ) ;
#4960=DIRECTION ( 'NONE',  ( -0.000000000000000000, -0.000000000000000000, -1.000000000000000000 ) ) ;
#4969=ORIENTED_EDGE ( 'NONE', *, *, #8636, .F. ) ;
#4976=CARTESIAN_POINT ( 'NONE',  ( -15.57266529552203416, 38.96488032230103471, 1.500000000000000000 ) ) ;
#4977=CARTESIAN_POINT ( 'NONE',  ( 16.52525247487311333, -14.36006998371588317, -1.500000000000000000 ) ) ;
#4985=ORIENTED_EDGE ( 'NONE', *, *, #15762, .T. ) ;
#4987=CARTESIAN_POINT ( 'NONE',  ( -4.100931858250860707, -19.90478481566557534, -1.500000000000000000 ) ) ;
#5008=CYLINDRICAL_SURFACE ( 'NONE', #12575, 2.898871837527151829 ) ;
#5011=EDGE_CURVE ( 'NONE', #7329, #6434, #27259, .T. ) ;
#5018=LINE ( 'NONE', #14375, #17850 ) ;
#5034=EDGE_CURVE ( 'NONE', #3349, #22024, #10832, .T. ) ;
#5049=ORIENTED_EDGE ( 'NONE', *, *, #26547, .T. ) ;
#5059=CARTESIAN_POINT ( 'NONE',  ( 8.260402557893151254, 8.184276679720483116, -1.500000000000000000 ) ) ;
#5072=EDGE_LOOP ( 'NONE', ( #23650, #17074, #10196, #11676 ) ) ;
#5097=CIRCLE ( 'NONE', #1113, 21.71568325578193637 ) ;
#5113=AXIS2_PLACEMENT_3D ( 'NONE', #24196, #5189, #8006 ) ;
#5114=VECTOR ( 'NONE', #18706, 1000.000000000000000 ) ;
#5121=( BOUNDED_SURFACE ( )  B_SPLINE_SURFACE ( 3, 1, ( 
 ( #19077, #19390 ),
 ( #28595, #12534 ),
 ( #14228, #663 ),
 ( #12065, #26094 ) ),
 .UNSPECIFIED., .F., .F., .F. ) 
 B_SPLINE_SURFACE_WITH_KNOTS ( ( 4, 4 ),
 ( 2, 2 ),
 ( 0.000000000000000000, 1.000000000000000000 ),
 ( 0.000000000000000000, 1.000000000000000000 ),
 .UNSPECIFIED. ) 
 GEOMETRIC_REPRESENTATION_ITEM ( )  RATIONAL_B_SPLINE_SURFACE ( (
 ( 1.000000000000000000, 1.000000000000000000),
 ( 0.8179194830933627092, 0.8179194830933627092),
 ( 0.8179194830933627092, 0.8179194830933627092),
 ( 1.000000000000000000, 1.000000000000000000) ) ) 
 REPRESENTATION_ITEM ( '' )  SURFACE ( )  );
#5146=VERTEX_POINT ( 'NONE', #10400 ) ;
#5153=CIRCLE ( 'NONE', #7146, 0.7441270634456903510 ) ;
#5156=CIRCLE ( 'NONE', #25089, 1.447898107987170890 ) ;
#5160=CARTESIAN_POINT ( 'NONE',  ( 3.118309183252346628, -17.14266753270391774, 1.500000000000000000 ) ) ;
#5172=EDGE_CURVE ( 'NONE', #2517, #27291, #16812, .T. ) ;
#5189=DIRECTION ( 'NONE',  ( -0.000000000000000000, 0.000000000000000000, 1.000000000000000000 ) ) ;
#5193=CARTESIAN_POINT ( 'NONE',  ( -14.41708049311053053, 17.22181377296911720, 1.500000000000000000 ) ) ;
#5195=APPLICATION_CONTEXT ( 'automotive_design' ) ;
#5197=ORIENTED_EDGE ( 'NONE', *, *, #2117, .F. ) ;
#5226=VERTEX_POINT ( 'NONE', #6326 ) ;
#5236=EDGE_CURVE ( 'NONE', #15112, #21717, #8365, .T. ) ;
#5239=EDGE_CURVE ( 'NONE', #26950, #3989, #374, .T. ) ;
#5250=CIRCLE ( 'NONE', #26664, 0.6002263538043648428 ) ;
#5251=CARTESIAN_POINT ( 'NONE',  ( 0.000000000000000000, 0.000000000000000000, 1.500000000000000000 ) ) ;
#5262=VERTEX_POINT ( 'NONE', #20058 ) ;
#5265=ORIENTED_EDGE ( 'NONE', *, *, #18963, .T. ) ;
#5279=VECTOR ( 'NONE', #8978, 1000.000000000000000 ) ;
#5295=CARTESIAN_POINT ( 'NONE',  ( -3.515970705488605130, -17.06554576617236307, 1.500000000000000000 ) ) ;
#5296=CARTESIAN_POINT ( 'NONE',  ( 28.34828976096171971, 29.18752572968384129, -1.500000000000000000 ) ) ;
#5304=CARTESIAN_POINT ( 'NONE',  ( 8.860628911697515875, 8.184276679720483116, -1.500000000000000000 ) ) ;
#5322=DIRECTION ( 'NONE',  ( -1.000000000000000000, 0.000000000000000000, 0.000000000000000000 ) ) ;
#5323=CARTESIAN_POINT ( 'NONE',  ( -19.54426622602688468, -37.07991288358296345, 1.499999999999999778 ) ) ;
#5333=CARTESIAN_POINT ( 'NONE',  ( 9.301547456646380496, 8.591538895647095941, 1.500000000000000000 ) ) ;
#5341=CIRCLE ( 'NONE', #25787, 1.447898107987198646 ) ;
#5344=CIRCLE ( 'NONE', #20289, 2.061368542273053883 ) ;
#5355=ORIENTED_EDGE ( 'NONE', *, *, #25009, .F. ) ;
#5368=CARTESIAN_POINT ( 'NONE',  ( 0.000000000000000000, 0.000000000000000000, -1.500000000000000000 ) ) ;
#5371=CARTESIAN_POINT ( 'NONE',  ( -4.163336342344337027E-14, -1.387778780781445676E-14, -1.500000000000000000 ) ) ;
#5378=ORIENTED_EDGE ( 'NONE', *, *, #13579, .T. ) ;
#5381=CARTESIAN_POINT ( 'NONE',  ( 0.000000000000000000, 0.000000000000000000, 1.500000000000000000 ) ) ;
#5387=ORIENTED_EDGE ( 'NONE', *, *, #5617, .F. ) ;
#5392=CARTESIAN_POINT ( 'NONE',  ( 3.221450758838616757, -1.621276839356792454, -1.500000000000000000 ) ) ;
#5408=FACE_OUTER_BOUND ( 'NONE', #13542, .T. ) ;
#5410=CARTESIAN_POINT ( 'NONE',  ( 16.65122935894595813, 13.93942108199718888, -1.500000000000000000 ) ) ;
#5411=CARTESIAN_POINT ( 'NONE',  ( -4.163336342344337027E-14, -1.387778780781445676E-14, 1.500000000000000000 ) ) ;
#5457=ORIENTED_EDGE ( 'NONE', *, *, #13187, .T. ) ;
#5471=ORIENTED_EDGE ( 'NONE', *, *, #13002, .F. ) ;
#5483=CARTESIAN_POINT ( 'NONE',  ( 0.000000000000000000, 0.000000000000000000, 1.500000000000000000 ) ) ;
#5494=DIRECTION ( 'NONE',  ( 0.000000000000000000, -0.000000000000000000, -1.000000000000000000 ) ) ;
#5510=DIRECTION ( 'NONE',  ( -1.000000000000000000, 0.000000000000000000, 0.000000000000000000 ) ) ;
#5523=CYLINDRICAL_SURFACE ( 'NONE', #9799, 0.7441270634457181066 ) ;
#5548=CARTESIAN_POINT ( 'NONE',  ( -13.93942108199721730, 16.65122935894503442, 1.500000000000000000 ) ) ;
#5554=DIRECTION ( 'NONE',  ( -0.000000000000000000, -0.000000000000000000, -1.000000000000000000 ) ) ;
#5581=EDGE_CURVE ( 'NONE', #24520, #13253, #5097, .T. ) ;
#5597=CARTESIAN_POINT ( 'NONE',  ( -6.414842543015754295, 17.06554576617236307, -1.500000000000000000 ) ) ;
#5605=DIRECTION ( 'NONE',  ( -0.000000000000000000, -0.000000000000000000, -1.000000000000000000 ) ) ;
#5606=CARTESIAN_POINT ( 'NONE',  ( 14.83584055149749759, 17.84153987719500734, -1.500000000000000000 ) ) ;
#5617=EDGE_CURVE ( 'NONE', #27291, #8486, #6075, .T. ) ;
#5629=CARTESIAN_POINT ( 'NONE',  ( 23.17581250239729940, 34.50630206824671831, 1.499999999999999778 ) ) ;
#5635=ORIENTED_EDGE ( 'NONE', *, *, #429, .T. ) ;
#5649=CARTESIAN_POINT ( 'NONE',  ( 9.675133109038689838, -8.168544852422947145, 1.500000000000000000 ) ) ;
#5650=DIRECTION ( 'NONE',  ( -0.000000000000000000, -0.000000000000000000, -1.000000000000000000 ) ) ;
#5685=DIRECTION ( 'NONE',  ( -0.4495526574063634095, 0.8932538319083086487, 0.000000000000000000 ) ) ;
#5698=VERTEX_POINT ( 'NONE', #1917 ) ;
#5702=LINE ( 'NONE', #15196, #4864 ) ;
#5714=ORIENTED_EDGE ( 'NONE', *, *, #23526, .T. ) ;
#5716=DIRECTION ( 'NONE',  ( 1.000000000000000000, 0.000000000000000000, 0.000000000000000000 ) ) ;
#5727=EDGE_CURVE ( 'NONE', #27254, #27382, #23492, .T. ) ;
#5731=CARTESIAN_POINT ( 'NONE',  ( -16.69721919944057831, 13.88429941593312122, 1.500000000000000000 ) ) ;
#5745=EDGE_CURVE ( 'NONE', #16359, #25738, #8953, .T. ) ;
#5760=CARTESIAN_POINT ( 'NONE',  ( 43.34097750826426676, -11.89502811014148698, -1.500000000000000444 ) ) ;
#5761=DIRECTION ( 'NONE',  ( -0.000000000000000000, -0.000000000000000000, -1.000000000000000000 ) ) ;
#5778=DIRECTION ( 'NONE',  ( 0.7416830501633135952, -0.6707505147970024284, 0.000000000000000000 ) ) ;
#5781=CIRCLE ( 'NONE', #14220, 2.898871837527149609 ) ;
#5788=FACE_OUTER_BOUND ( 'NONE', #23786, .T. ) ;
#5796=DIRECTION ( 'NONE',  ( 1.000000000000000000, 0.000000000000000000, 0.000000000000000000 ) ) ;
#5799=VECTOR ( 'NONE', #17977, 1000.000000000000000 ) ;
#5821=MECHANICAL_DESIGN_GEOMETRIC_PRESENTATION_REPRESENTATION('',(#18749),#19698);
#5836=CARTESIAN_POINT ( 'NONE',  ( 16.52525247487311333, -14.36006998371588317, 1.500000000000000000 ) ) ;
#5848=CARTESIAN_POINT ( 'NONE',  ( 26.73000961532937225, -9.331429872129930914, 1.500000000000000000 ) ) ;
#5866=CARTESIAN_POINT ( 'NONE',  ( 26.36764545593179676, 31.31467416275351923, -1.500000000000000000 ) ) ;
#5872=DIRECTION ( 'NONE',  ( -0.000000000000000000, -0.000000000000000000, -1.000000000000000000 ) ) ;
#5889=EDGE_LOOP ( 'NONE', ( #29000, #27416, #18759, #20539 ) ) ;
#5919=DIRECTION ( 'NONE',  ( 1.000000000000000000, 0.000000000000000000, 0.000000000000000000 ) ) ;
#5926=ORIENTED_EDGE ( 'NONE', *, *, #22730, .F. ) ;
#5928=ADVANCED_FACE ( 'NONE', ( #23891 ), #27131, .F. ) ;
#5945=VECTOR ( 'NONE', #5685, 1000.000000000000000 ) ;
#5949=EDGE_CURVE ( 'NONE', #1513, #19394, #7957, .T. ) ;
#5996=ORIENTED_EDGE ( 'NONE', *, *, #14149, .T. ) ;
#6001=DIRECTION ( 'NONE',  ( 1.000000000000000000, 0.000000000000000000, 0.000000000000000000 ) ) ;
#6004=DIRECTION ( 'NONE',  ( 0.000000000000000000, -0.000000000000000000, -1.000000000000000000 ) ) ;
#6006=EDGE_LOOP ( 'NONE', ( #59, #25868, #11734, #28083 ) ) ;
#6010=DIRECTION ( 'NONE',  ( -0.000000000000000000, -0.000000000000000000, -1.000000000000000000 ) ) ;
#6018=CARTESIAN_POINT ( 'NONE',  ( 17.79239818699415920, 14.89473990422378158, 1.500000000000000000 ) ) ;
#6019=DIRECTION ( 'NONE',  ( 0.000000000000000000, -0.000000000000000000, -1.000000000000000000 ) ) ;
#6039=VERTEX_POINT ( 'NONE', #2291 ) ;
#6050=VERTEX_POINT ( 'NONE', #2002 ) ;
#6052=AXIS2_PLACEMENT_3D ( 'NONE', #28185, #2456, #9315 ) ;
#6071=DIRECTION ( 'NONE',  ( 1.000000000000000000, 0.000000000000000000, 0.000000000000000000 ) ) ;
#6075=CIRCLE ( 'NONE', #28005, 0.7441270634457198829 ) ;
#6105=DIRECTION ( 'NONE',  ( -0.000000000000000000, -0.000000000000000000, -1.000000000000000000 ) ) ;
#6107=EDGE_LOOP ( 'NONE', ( #11555, #27093, #27569, #3308 ) ) ;
#6112=EDGE_LOOP ( 'NONE', ( #17352, #23201, #18330, #6297 ) ) ;
#6118=AXIS2_PLACEMENT_3D ( 'NONE', #10274, #8256, #12782 ) ;
#6127=DIRECTION ( 'NONE',  ( -1.000000000000000000, 0.000000000000000000, 0.000000000000000000 ) ) ;
#6128=CARTESIAN_POINT ( 'NONE',  ( 9.216505592218814158, -7.781333699927420966, 1.500000000000000000 ) ) ;
#6132=EDGE_CURVE ( 'NONE', #5146, #9927, #22030, .T. ) ;
#6155=EDGE_CURVE ( 'NONE', #12669, #27956, #19923, .T. ) ;
#6161=EDGE_CURVE ( 'NONE', #27927, #24914, #17718, .T. ) ;
#6167=EDGE_CURVE ( 'NONE', #22024, #24302, #568, .T. ) ;
#6179=CARTESIAN_POINT ( 'NONE',  ( 3.221450758838616757, 1.621276839356792454, 1.500000000000000000 ) ) ;
#6201=ORIENTED_EDGE ( 'NONE', *, *, #17435, .F. ) ;
#6222=DIRECTION ( 'NONE',  ( 1.000000000000000000, 0.000000000000000000, 0.000000000000000000 ) ) ;
#6223=CARTESIAN_POINT ( 'NONE',  ( -6.414842543015754295, -17.06554576617236307, 1.500000000000000000 ) ) ;
#6235=ORIENTED_EDGE ( 'NONE', *, *, #16442, .F. ) ;
#6256=CARTESIAN_POINT ( 'NONE',  ( -30.75232512042845556, -9.966982604840850968, 1.500000000000000000 ) ) ;
#6260=( NAMED_UNIT ( * ) SI_UNIT ( $, .STERADIAN. ) SOLID_ANGLE_UNIT ( ) );
#6270=AXIS2_PLACEMENT_3D ( 'NONE', #3588, #8122, #12799 ) ;
#6278=DIRECTION ( 'NONE',  ( -0.000000000000000000, -0.000000000000000000, -1.000000000000000000 ) ) ;
#6279=CARTESIAN_POINT ( 'NONE',  ( 24.03057240117691862, 26.57182937991349903, -1.500000000000000000 ) ) ;
#6282=CARTESIAN_POINT ( 'NONE',  ( 0.000000000000000000, -5.590849009245238754, 1.500000000000000000 ) ) ;
#6283=CARTESIAN_POINT ( 'NONE',  ( -4.163336342344337027E-14, -1.387778780781445676E-14, -1.500000000000000000 ) ) ;
#6285=VERTEX_POINT ( 'NONE', #29280 ) ;
#6293=AXIS2_PLACEMENT_3D ( 'NONE', #17415, #21925, #19588 ) ;
#6297=ORIENTED_EDGE ( 'NONE', *, *, #23476, .T. ) ;
#6298=DIRECTION ( 'NONE',  ( -0.000000000000000000, 0.000000000000000000, 1.000000000000000000 ) ) ;
#6323=DIRECTION ( 'NONE',  ( -0.000000000000000000, 0.000000000000000000, 1.000000000000000000 ) ) ;
#6326=CARTESIAN_POINT ( 'NONE',  ( 26.36764545593179676, 31.31467416275351923, -1.500000000000000000 ) ) ;
#6349=ADVANCED_FACE ( 'NONE', ( #1202 ), #24904, .F. ) ;
#6358=CARTESIAN_POINT ( 'NONE',  ( -1.073881485057738949, -0.9711784013061123266, 1.500000000000000000 ) ) ;
#6367=DIRECTION ( 'NONE',  ( -1.000000000000000000, 0.000000000000000000, 0.000000000000000000 ) ) ;
#6374=CARTESIAN_POINT ( 'NONE',  ( 1.073881485057758711, 0.9711784013061475207, -1.500000000000000000 ) ) ;
#6387=ORIENTED_EDGE ( 'NONE', *, *, #25009, .T. ) ;
#6403=EDGE_CURVE ( 'NONE', #16254, #4466, #30637, .T. ) ;
#6405=CARTESIAN_POINT ( 'NONE',  ( -17.22181377296915272, -14.41708049311147555, 1.500000000000000000 ) ) ;
#6417=ORIENTED_EDGE ( 'NONE', *, *, #907, .T. ) ;
#6434=VERTEX_POINT ( 'NONE', #2422 ) ;
#6438=UNCERTAINTY_MEASURE_WITH_UNIT (LENGTH_MEASURE( 1.000000000000000082E-05 ), #1443, 'distance_accuracy_value', 'NONE');
#6449=CARTESIAN_POINT ( 'NONE',  ( -24.03057240117691862, 26.57182937991349903, 1.500000000000000000 ) ) ;
#6461=DIRECTION ( 'NONE',  ( -0.000000000000000000, 0.000000000000000000, 1.000000000000000000 ) ) ;
#6482=LINE ( 'NONE', #3992, #14210 ) ;
#6501=CIRCLE ( 'NONE', #27374, 12.66227964008302287 ) ;
#6540=ORIENTED_EDGE ( 'NONE', *, *, #16064, .F. ) ;
#6547=CARTESIAN_POINT ( 'NONE',  ( 22.95669091611932089, -27.54300778121948312, -1.500000000000000000 ) ) ;
#6548=EDGE_CURVE ( 'NONE', #3169, #26376, #14885, .T. ) ;
#6552=EDGE_CURVE ( 'NONE', #18859, #1513, #24234, .T. ) ;
#6553=CYLINDRICAL_SURFACE ( 'NONE', #24099, 0.6002263538043630664 ) ;
#6585=ORIENTED_EDGE ( 'NONE', *, *, #10687, .T. ) ;
#6591=AXIS2_PLACEMENT_3D ( 'NONE', #25782, #4411, #9407 ) ;
#6592=DIRECTION ( 'NONE',  ( -0.6707505147970090897, 0.7416830501633074890, 0.000000000000000000 ) ) ;
#6600=VERTEX_POINT ( 'NONE', #24546 ) ;
#6615=ORIENTED_EDGE ( 'NONE', *, *, #17370, .F. ) ;
#6631=CARTESIAN_POINT ( 'NONE',  ( -4.163336342344337027E-14, -1.387778780781445676E-14, 1.500000000000000000 ) ) ;
#6639=ORIENTED_EDGE ( 'NONE', *, *, #9960, .F. ) ;
#6660=DIRECTION ( 'NONE',  ( -0.000000000000000000, -0.000000000000000000, -1.000000000000000000 ) ) ;
#6665=CARTESIAN_POINT ( 'NONE',  ( 26.36764545593177544, -31.31467416275353344, 1.500000000000000000 ) ) ;
#6666=AXIS2_PLACEMENT_3D ( 'NONE', #19605, #19926, #26953 ) ;
#6709=EDGE_CURVE ( 'NONE', #21157, #10630, #22054, .T. ) ;
#6720=EDGE_CURVE ( 'NONE', #19394, #13900, #2153, .T. ) ;
#6739=DIRECTION ( 'NONE',  ( -0.000000000000000000, 0.000000000000000000, 1.000000000000000000 ) ) ;
#6745=AXIS2_PLACEMENT_3D ( 'NONE', #8707, #16338, #6367 ) ;
#6747=VERTEX_POINT ( 'NONE', #8342 ) ;
#6759=AXIS2_PLACEMENT_3D ( 'NONE', #21371, #9994, #2656 ) ;
#6766=DIRECTION ( 'NONE',  ( -0.000000000000000000, -0.000000000000000000, -1.000000000000000000 ) ) ;
#6787=VERTEX_POINT ( 'NONE', #4716 ) ;
#6799=AXIS2_PLACEMENT_3D ( 'NONE', #15837, #13669, #4138 ) ;
#6807=DIRECTION ( 'NONE',  ( -0.000000000000000000, 0.000000000000000000, 1.000000000000000000 ) ) ;
#6819=VERTEX_POINT ( 'NONE', #19064 ) ;
#6830=FACE_OUTER_BOUND ( 'NONE', #21336, .T. ) ;
#6841=VERTEX_POINT ( 'NONE', #7058 ) ;
#6842=ORIENTED_EDGE ( 'NONE', *, *, #9430, .T. ) ;
#6848=AXIS2_PLACEMENT_3D ( 'NONE', #6282, #18463, #1469 ) ;
#6854=EDGE_CURVE ( 'NONE', #7845, #13900, #25639, .T. ) ;
#6863=CYLINDRICAL_SURFACE ( 'NONE', #26768, 21.71568325578263625 ) ;
#6882=AXIS2_PLACEMENT_3D ( 'NONE', #27040, #20008, #10185 ) ;
#6893=LINE ( 'NONE', #26, #29262 ) ;
#6896=ORIENTED_EDGE ( 'NONE', *, *, #29594, .T. ) ;
#6915=EDGE_CURVE ( 'NONE', #12408, #8486, #8625, .T. ) ;
#6922=DIRECTION ( 'NONE',  ( 1.000000000000000000, 0.000000000000000000, 0.000000000000000000 ) ) ;
#6925=EDGE_LOOP ( 'NONE', ( #30690, #28766, #20898, #18247, #21594 ) ) ;
#6930=EDGE_CURVE ( 'NONE', #8512, #26677, #26564, .T. ) ;
#6945=( BOUNDED_CURVE ( )  B_SPLINE_CURVE ( 3, ( #19581, #28792, #3356, #703 ),
 .UNSPECIFIED., .F., .T. ) 
 B_SPLINE_CURVE_WITH_KNOTS ( ( 4, 4 ),
 ( 3.552344893626886879, 3.884040399493172036 ),
 .UNSPECIFIED. ) 
 CURVE ( )  GEOMETRIC_REPRESENTATION_ITEM ( )  RATIONAL_B_SPLINE_CURVE ( ( 1.000000000000000000, 0.9908525036704132205, 0.9908525036704132205, 1.000000000000000000 ) ) 
 REPRESENTATION_ITEM ( '' )  );
#6956=DIRECTION ( 'NONE',  ( -0.000000000000000000, 0.000000000000000000, 1.000000000000000000 ) ) ;
#6957=FACE_OUTER_BOUND ( 'NONE', #24210, .T. ) ;
#6962=EDGE_CURVE ( 'NONE', #24520, #3590, #17589, .T. ) ;
#6974=VERTEX_POINT ( 'NONE', #11105 ) ;
#7001=EDGE_LOOP ( 'NONE', ( #8009, #6417, #3907, #18478 ) ) ;
#7011=PLANE ( 'NONE',  #27825 ) ;
#7018=ORIENTED_EDGE ( 'NONE', *, *, #8039, .F. ) ;
#7025=CARTESIAN_POINT ( 'NONE',  ( -11.21147646446735102, 30.29926891764210595, 1.500000000000000000 ) ) ;
#7027=VERTEX_POINT ( 'NONE', #17978 ) ;
#7037=CARTESIAN_POINT ( 'NONE',  ( 28.34828976096172681, -29.18752572968383419, -1.500000000000000000 ) ) ;
#7053=DIRECTION ( 'NONE',  ( 1.000000000000000000, 0.000000000000000000, 0.000000000000000000 ) ) ;
#7057=EDGE_CURVE ( 'NONE', #24048, #24781, #5156, .T. ) ;
#7058=CARTESIAN_POINT ( 'NONE',  ( -23.20393738267338790, 0.000000000000000000, 1.500000000000000000 ) ) ;
#7065=VERTEX_POINT ( 'NONE', #27637 ) ;
#7069=CARTESIAN_POINT ( 'NONE',  ( -11.21147646446735102, -30.29926891764210595, 1.500000000000000000 ) ) ;
#7071=ORIENTED_EDGE ( 'NONE', *, *, #20062, .T. ) ;
#7075=EDGE_CURVE ( 'NONE', #12516, #28935, #3617, .T. ) ;
#7103=VERTEX_POINT ( 'NONE', #16226 ) ;
#7104=DIRECTION ( 'NONE',  ( 0.000000000000000000, -0.000000000000000000, -1.000000000000000000 ) ) ;
#7107=CARTESIAN_POINT ( 'NONE',  ( -1.073881485057447405, -0.9711784013058452070, 1.500000000000000000 ) ) ;
#7124=EDGE_CURVE ( 'NONE', #27347, #13900, #23234, .T. ) ;
#7129=SHAPE_REPRESENTATION ( 'Front & Rear Ported Pressure', ( #7396 ), #910 ) ;
#7140=EDGE_CURVE ( 'NONE', #1105, #16393, #25583, .T. ) ;
#7146=AXIS2_PLACEMENT_3D ( 'NONE', #25096, #30235, #5919 ) ;
#7149=ORIENTED_EDGE ( 'NONE', *, *, #27118, .T. ) ;
#7150=DIRECTION ( 'NONE',  ( -1.000000000000000000, 0.000000000000000000, 0.000000000000000000 ) ) ;
#7159=AXIS2_PLACEMENT_3D ( 'NONE', #26183, #23382, #14023 ) ;
#7174=ORIENTED_EDGE ( 'NONE', *, *, #27712, .T. ) ;
#7180=CARTESIAN_POINT ( 'NONE',  ( 17.84153987719590972, -14.83584055149750114, -1.500000000000000000 ) ) ;
#7216=CARTESIAN_POINT ( 'NONE',  ( -26.44644203219470668, 9.801837641955994940, -1.500000000000000000 ) ) ;
#7229=CARTESIAN_POINT ( 'NONE',  ( 30.75232512042845556, -9.966982604840845639, -1.500000000000000000 ) ) ;
#7246=DIRECTION ( 'NONE',  ( 0.7416830501633145944, 0.6707505147970012072, -0.000000000000000000 ) ) ;
#7252=DIRECTION ( 'NONE',  ( 0.6707505147970010961, -0.7416830501633147055, 0.000000000000000000 ) ) ;
#7258=CIRCLE ( 'NONE', #24685, 11.46182693247435935 ) ;
#7261=EDGE_LOOP ( 'NONE', ( #23466, #16193, #19574, #21807 ) ) ;
#7262=LINE ( 'NONE', #19270, #7315 ) ;
#7277=EDGE_CURVE ( 'NONE', #23361, #21731, #16384, .T. ) ;
#7278=DIRECTION ( 'NONE',  ( -0.000000000000000000, -0.000000000000000000, -1.000000000000000000 ) ) ;
#7286=ORIENTED_EDGE ( 'NONE', *, *, #6854, .T. ) ;
#7298=CIRCLE ( 'NONE', #9341, 0.6002263538043630664 ) ;
#7303=DIRECTION ( 'NONE',  ( 1.000000000000000000, 1.776356839400250465E-15, 0.000000000000000000 ) ) ;
#7306=DIRECTION ( 'NONE',  ( -0.7416830501633076000, -0.6707505147970089787, 0.000000000000000000 ) ) ;
#7310=EDGE_LOOP ( 'NONE', ( #30547, #8233, #22839, #4533 ) ) ;
#7315=VECTOR ( 'NONE', #18820, 1000.000000000000000 ) ;
#7328=FACE_BOUND ( 'NONE', #2554, .T. ) ;
#7329=VERTEX_POINT ( 'NONE', #7180 ) ;
#7336=CARTESIAN_POINT ( 'NONE',  ( 0.000000000000000000, 0.000000000000000000, 1.500000000000000000 ) ) ;
#7374=VECTOR ( 'NONE', #27537, 1000.000000000000000 ) ;
#7377=CIRCLE ( 'NONE', #24804, 2.898871837527151385 ) ;
#7384=EDGE_LOOP ( 'NONE', ( #19751, #23047, #3480, #3741 ) ) ;
#7388=CARTESIAN_POINT ( 'NONE',  ( 26.83043119477639138, -8.695877139419035728, 1.500000000000000000 ) ) ;
#7396=AXIS2_PLACEMENT_3D ( 'NONE', #9486, #28514, #21014 ) ;
#7412=CARTESIAN_POINT ( 'NONE',  ( 28.79137815760242702, -9.331429872129930914, 1.500000000000000000 ) ) ;
#7416=ORIENTED_EDGE ( 'NONE', *, *, #17785, .T. ) ;
#7435=EDGE_CURVE ( 'NONE', #3590, #6841, #4158, .T. ) ;
#7437=CARTESIAN_POINT ( 'NONE',  ( 25.10445388623454477, 25.60065097860747585, 1.500000000000000000 ) ) ;
#7456=VERTEX_POINT ( 'NONE', #27604 ) ;
#7457=DIRECTION ( 'NONE',  ( -0.6707505147970090897, -0.7416830501633074890, 0.000000000000000000 ) ) ;
#7461=EDGE_CURVE ( 'NONE', #7103, #6285, #24628, .T. ) ;
#7471=FACE_OUTER_BOUND ( 'NONE', #3799, .T. ) ;
#7492=DIRECTION ( 'NONE',  ( -1.000000000000000000, 0.000000000000000000, 0.000000000000000000 ) ) ;
#7505=CARTESIAN_POINT ( 'NONE',  ( 25.10445388623454477, -25.60065097860747585, -1.500000000000000000 ) ) ;
#7508=ORIENTED_EDGE ( 'NONE', *, *, #6167, .T. ) ;
#7535=CARTESIAN_POINT ( 'NONE',  ( -4.163336342344337027E-14, -1.387778780781445676E-14, 1.500000000000000000 ) ) ;
#7539=VECTOR ( 'NONE', #13091, 1000.000000000000000 ) ;
#7544=EDGE_LOOP ( 'NONE', ( #23228, #1360, #23628, #15707 ) ) ;
#7560=CIRCLE ( 'NONE', #10050, 2.898871837527149609 ) ;
#7567=DIRECTION ( 'NONE',  ( -0.000000000000000000, -0.000000000000000000, -1.000000000000000000 ) ) ;
#7569=ORIENTED_EDGE ( 'NONE', *, *, #18561, .T. ) ;
#7570=EDGE_LOOP ( 'NONE', ( #21258, #11374, #24118, #10423 ) ) ;
#7572=ADVANCED_FACE ( 'NONE', ( #6957 ), #19260, .F. ) ;
#7593=CARTESIAN_POINT ( 'NONE',  ( 16.69721919944051791, -13.88429941593332551, 1.500000000000000000 ) ) ;
#7610=VECTOR ( 'NONE', #10942, 1000.000000000000000 ) ;
#7631=PRODUCT_DEFINITION ( 'UNKNOWN', '', #17893, #3913 ) ;
#7637=ORIENTED_EDGE ( 'NONE', *, *, #1997, .T. ) ;
#7640=CARTESIAN_POINT ( 'NONE',  ( 28.34828976096171971, -29.18752572968383419, -1.500000000000000000 ) ) ;
#7665=DIRECTION ( 'NONE',  ( -0.000000000000000000, 0.000000000000000000, 1.000000000000000000 ) ) ;
#7675=EDGE_CURVE ( 'NONE', #29550, #19640, #29554, .T. ) ;
#7678=LINE ( 'NONE', #21225, #16785 ) ;
#7680=ORIENTED_EDGE ( 'NONE', *, *, #8636, .T. ) ;
#7691=EDGE_CURVE ( 'NONE', #28435, #24290, #21909, .T. ) ;
#7733=ORIENTED_EDGE ( 'NONE', *, *, #22939, .T. ) ;
#7789=ORIENTED_EDGE ( 'NONE', *, *, #14737, .F. ) ;
#7807=DIRECTION ( 'NONE',  ( -0.000000000000000000, -0.000000000000000000, -1.000000000000000000 ) ) ;
#7827=DIRECTION ( 'NONE',  ( 0.000000000000000000, -0.000000000000000000, -1.000000000000000000 ) ) ;
#7845=VERTEX_POINT ( 'NONE', #15657 ) ;
#7849=EDGE_CURVE ( 'NONE', #24302, #9342, #24016, .T. ) ;
#7850=DIRECTION ( 'NONE',  ( -0.000000000000000000, 0.000000000000000000, 1.000000000000000000 ) ) ;
#7869=ORIENTED_EDGE ( 'NONE', *, *, #21854, .T. ) ;
#7876=DIRECTION ( 'NONE',  ( -0.000000000000000000, -0.000000000000000000, -1.000000000000000000 ) ) ;
#7904=FACE_OUTER_BOUND ( 'NONE', #23645, .T. ) ;
#7913=DIRECTION ( 'NONE',  ( -0.000000000000000000, -0.000000000000000000, -1.000000000000000000 ) ) ;
#7915=DIRECTION ( 'NONE',  ( -0.000000000000000000, 0.000000000000000000, 1.000000000000000000 ) ) ;
#7925=ORIENTED_EDGE ( 'NONE', *, *, #7140, .F. ) ;
#7942=AXIS2_PLACEMENT_3D ( 'NONE', #16000, #25668, #4288 ) ;
#7957=LINE ( 'NONE', #2536, #12094 ) ;
#7958=LINE ( 'NONE', #1510, #1938 ) ;
#7967=LINE ( 'NONE', #17473, #21626 ) ;
#7973=AXIS2_PLACEMENT_3D ( 'NONE', #9489, #21641, #7303 ) ;
#7978=EDGE_LOOP ( 'NONE', ( #10179, #15294, #570, #28682 ) ) ;
#7987=DIRECTION ( 'NONE',  ( -0.000000000000000000, -0.000000000000000000, -1.000000000000000000 ) ) ;
#7989=LINE ( 'NONE', #17332, #12909 ) ;
#7992=CYLINDRICAL_SURFACE ( 'NONE', #2841, 12.66227964008302287 ) ;
#7993=DIRECTION ( 'NONE',  ( -0.000000000000000000, 0.000000000000000000, 1.000000000000000000 ) ) ;
#8002=AXIS2_PLACEMENT_3D ( 'NONE', #7535, #2385, #4877 ) ;
#8006=DIRECTION ( 'NONE',  ( 1.000000000000000000, 0.000000000000000000, 0.000000000000000000 ) ) ;
#8009=ORIENTED_EDGE ( 'NONE', *, *, #27729, .T. ) ;
#8011=CARTESIAN_POINT ( 'NONE',  ( -1.073881485057738949, 0.9711784013061123266, 1.500000000000000000 ) ) ;
#8013=ORIENTED_EDGE ( 'NONE', *, *, #18029, .T. ) ;
#8016=VERTEX_POINT ( 'NONE', #30017 ) ;
#8039=EDGE_CURVE ( 'NONE', #1352, #30322, #26533, .T. ) ;
#8049=EDGE_CURVE ( 'NONE', #9427, #24441, #14395, .T. ) ;
#8071=LINE ( 'NONE', #29730, #11786 ) ;
#8072=DIRECTION ( 'NONE',  ( -0.000000000000000000, 0.000000000000000000, 1.000000000000000000 ) ) ;
#8075=ORIENTED_EDGE ( 'NONE', *, *, #29575, .T. ) ;
#8122=DIRECTION ( 'NONE',  ( 0.000000000000000000, -0.000000000000000000, -1.000000000000000000 ) ) ;
#8135=DIRECTION ( 'NONE',  ( -1.000000000000000000, 0.000000000000000000, 0.000000000000000000 ) ) ;
#8136=( BOUNDED_CURVE ( )  B_SPLINE_CURVE ( 3, ( #21020, #18552, #28056, #30542 ),
 .UNSPECIFIED., .F., .T. ) 
 B_SPLINE_CURVE_WITH_KNOTS ( ( 4, 4 ),
 ( 0.4107522400370940407, 0.7424477459033789195 ),
 .UNSPECIFIED. ) 
 CURVE ( )  GEOMETRIC_REPRESENTATION_ITEM ( )  RATIONAL_B_SPLINE_CURVE ( ( 1.000000000000000000, 0.9908525036704132205, 0.9908525036704132205, 1.000000000000000000 ) ) 
 REPRESENTATION_ITEM ( '' )  );
#8155=VECTOR ( 'NONE', #16223, 1000.000000000000000 ) ;
#8175=ORIENTED_EDGE ( 'NONE', *, *, #11480, .T. ) ;
#8189=ORIENTED_EDGE ( 'NONE', *, *, #30, .T. ) ;
#8197=EDGE_CURVE ( 'NONE', #12669, #19397, #9100, .T. ) ;
#8203=EDGE_CURVE ( 'NONE', #25490, #11996, #29024, .T. ) ;
#8212=AXIS2_PLACEMENT_3D ( 'NONE', #8660, #29557, #24881 ) ;
#8219=ORIENTED_EDGE ( 'NONE', *, *, #907, .F. ) ;
#8228=ORIENTED_EDGE ( 'NONE', *, *, #12895, .F. ) ;
#8233=ORIENTED_EDGE ( 'NONE', *, *, #450, .F. ) ;
#8239=CARTESIAN_POINT ( 'NONE',  ( 43.34097750826427387, 11.89502811014146033, 1.500000000000000000 ) ) ;
#8256=DIRECTION ( 'NONE',  ( -0.000000000000000000, -0.000000000000000000, -1.000000000000000000 ) ) ;
#8259=CIRCLE ( 'NONE', #25687, 1.447898107987198646 ) ;
#8275=EDGE_CURVE ( 'NONE', #8512, #8763, #28985, .T. ) ;
#8291=ORIENTED_EDGE ( 'NONE', *, *, #19493, .F. ) ;
#8292=DIRECTION ( 'NONE',  ( -1.000000000000000000, 0.000000000000000000, 0.000000000000000000 ) ) ;
#8309=VERTEX_POINT ( 'NONE', #26498 ) ;
#8320=( BOUNDED_CURVE ( )  B_SPLINE_CURVE ( 3, ( #17845, #29687, #27362, #10354 ),
 .UNSPECIFIED., .F., .T. ) 
 B_SPLINE_CURVE_WITH_KNOTS ( ( 4, 4 ),
 ( 3.552344893626886879, 3.884040399493172036 ),
 .UNSPECIFIED. ) 
 CURVE ( )  GEOMETRIC_REPRESENTATION_ITEM ( )  RATIONAL_B_SPLINE_CURVE ( ( 1.000000000000000000, 0.9908525036704132205, 0.9908525036704132205, 1.000000000000000000 ) ) 
 REPRESENTATION_ITEM ( '' )  );
#8333=DIRECTION ( 'NONE',  ( -0.000000000000000000, -0.000000000000000000, -1.000000000000000000 ) ) ;
#8342=CARTESIAN_POINT ( 'NONE',  ( 16.69721919944051791, -13.88429941593332551, -1.500000000000000000 ) ) ;
#8355=ORIENTED_EDGE ( 'NONE', *, *, #6161, .T. ) ;
#8357=CIRCLE ( 'NONE', #19297, 21.71568325578193637 ) ;
#8364=FACE_OUTER_BOUND ( 'NONE', #20785, .T. ) ;
#8365=CIRCLE ( 'NONE', #3365, 20.32284676574536064 ) ;
#8369=CARTESIAN_POINT ( 'NONE',  ( -30.31220697679117393, 11.23460505553742550, 1.500000000000000000 ) ) ;
#8372=DIRECTION ( 'NONE',  ( 1.000000000000000000, 0.000000000000000000, 0.000000000000000000 ) ) ;
#8386=ORIENTED_EDGE ( 'NONE', *, *, #450, .T. ) ;
#8397=CIRCLE ( 'NONE', #6882, 0.7441270634456903510 ) ;
#8400=VERTEX_POINT ( 'NONE', #4977 ) ;
#8404=ORIENTED_EDGE ( 'NONE', *, *, #18029, .F. ) ;
#8446=EDGE_LOOP ( 'NONE', ( #17702, #30394, #25882, #28951 ) ) ;
#8450=EDGE_LOOP ( 'NONE', ( #26012, #28936, #18670, #17136 ) ) ;
#8462=ORIENTED_EDGE ( 'NONE', *, *, #24018, .T. ) ;
#8473=LINE ( 'NONE', #24509, #5799 ) ;
#8474=DIRECTION ( 'NONE',  ( -0.000000000000000000, 0.000000000000000000, 1.000000000000000000 ) ) ;
#8486=VERTEX_POINT ( 'NONE', #10737 ) ;
#8512=VERTEX_POINT ( 'NONE', #8711 ) ;
#8519=CARTESIAN_POINT ( 'NONE',  ( -11.21147646446735102, 30.29926891764210595, -1.500000000000000000 ) ) ;
#8530=CARTESIAN_POINT ( 'NONE',  ( 0.000000000000000000, 0.000000000000000000, 1.500000000000000000 ) ) ;
#8542=ORIENTED_EDGE ( 'NONE', *, *, #25401, .T. ) ;
#8549=ORIENTED_EDGE ( 'NONE', *, *, #15887, .F. ) ;
#8560=CARTESIAN_POINT ( 'NONE',  ( 28.34828976096172681, 29.18752572968383419, 1.500000000000000000 ) ) ;
#8570=DIRECTION ( 'NONE',  ( 1.000000000000000000, 0.000000000000000000, 0.000000000000000000 ) ) ;
#8572=DIRECTION ( 'NONE',  ( -0.000000000000000000, 0.000000000000000000, 1.000000000000000000 ) ) ;
#8575=ORIENTED_EDGE ( 'NONE', *, *, #6930, .T. ) ;
#8576=EDGE_LOOP ( 'NONE', ( #1205, #18432, #28252, #21161, #25804, #12163 ) ) ;
#8590=CARTESIAN_POINT ( 'NONE',  ( 19.54426622602689179, 37.07991288358296345, 1.499999999999999778 ) ) ;
#8612=DIRECTION ( 'NONE',  ( 1.000000000000000000, 0.000000000000000000, 0.000000000000000000 ) ) ;
#8625=CIRCLE ( 'NONE', #142, 21.71568325578263625 ) ;
#8632=CYLINDRICAL_SURFACE ( 'NONE', #18496, 14.52510309069105965 ) ;
#8636=EDGE_CURVE ( 'NONE', #26988, #10421, #4554, .T. ) ;
#8641=ADVANCED_FACE ( 'NONE', ( #14288 ), #11808, .T. ) ;
#8649=VECTOR ( 'NONE', #19035, 1000.000000000000000 ) ;
#8660=CARTESIAN_POINT ( 'NONE',  ( -4.163336342344337027E-14, -1.387778780781445676E-14, 1.500000000000000000 ) ) ;
#8665=CARTESIAN_POINT ( 'NONE',  ( 22.58267429318974706, -26.57182937991349903, -1.500000000000000000 ) ) ;
#8670=AXIS2_PLACEMENT_3D ( 'NONE', #15815, #18477, #6001 ) ;
#8688=AXIS2_PLACEMENT_3D ( 'NONE', #2773, #12599, #3386 ) ;
#8706=VECTOR ( 'NONE', #4960, 1000.000000000000000 ) ;
#8707=CARTESIAN_POINT ( 'NONE',  ( -4.163336342344337027E-14, -1.387778780781445676E-14, 1.500000000000000000 ) ) ;
#8711=CARTESIAN_POINT ( 'NONE',  ( 13.88429941593329531, 16.69721919943964039, 1.500000000000000000 ) ) ;
#8731=EDGE_LOOP ( 'NONE', ( #25889, #25910, #26551, #26896 ) ) ;
#8754=EDGE_CURVE ( 'NONE', #3343, #25145, #28038, .T. ) ;
#8763=VERTEX_POINT ( 'NONE', #25698 ) ;
#8780=DIRECTION ( 'NONE',  ( -0.000000000000000000, -0.000000000000000000, -1.000000000000000000 ) ) ;
#8808=VERTEX_POINT ( 'NONE', #1078 ) ;
#8846=VERTEX_POINT ( 'NONE', #11946 ) ;
#8870=LINE ( 'NONE', #3568, #7539 ) ;
#8924=CARTESIAN_POINT ( 'NONE',  ( -3.515970705488605130, -17.06554576617236307, 1.500000000000000000 ) ) ;
#8932=ORIENTED_EDGE ( 'NONE', *, *, #23604, .F. ) ;
#8944=DIRECTION ( 'NONE',  ( 1.000000000000000000, 0.000000000000000000, 0.000000000000000000 ) ) ;
#8953=LINE ( 'NONE', #18469, #11069 ) ;
#8963=ORIENTED_EDGE ( 'NONE', *, *, #10536, .F. ) ;
#8965=DIRECTION ( 'NONE',  ( 1.000000000000000000, -2.890115478905172036E-15, 0.000000000000000000 ) ) ;
#8978=DIRECTION ( 'NONE',  ( -0.000000000000000000, -0.000000000000000000, -1.000000000000000000 ) ) ;
#8979=ADVANCED_FACE ( 'NONE', ( #4746 ), #16754, .T. ) ;
#8988=ADVANCED_FACE ( 'NONE', ( #22048 ), #19879, .F. ) ;
#8993=VERTEX_POINT ( 'NONE', #12558 ) ;
#8997=DIRECTION ( 'NONE',  ( 1.000000000000000000, 0.000000000000000000, 0.000000000000000000 ) ) ;
#9012=CARTESIAN_POINT ( 'NONE',  ( 22.95669091611932089, -27.54300778121948312, 1.500000000000000000 ) ) ;
#9034=AXIS2_PLACEMENT_3D ( 'NONE', #22191, #29220, #27192 ) ;
#9044=CARTESIAN_POINT ( 'NONE',  ( 0.000000000000000000, 0.000000000000000000, 1.500000000000000000 ) ) ;
#9045=EDGE_CURVE ( 'NONE', #2551, #19699, #13802, .T. ) ;
#9047=ORIENTED_EDGE ( 'NONE', *, *, #8203, .F. ) ;
#9063=AXIS2_PLACEMENT_3D ( 'NONE', #12155, #9813, #9197 ) ;
#9083=CARTESIAN_POINT ( 'NONE',  ( -15.16120755655624741, 17.22181377296911720, -1.500000000000000000 ) ) ;
#9100=CIRCLE ( 'NONE', #5113, 10.00000000000000000 ) ;
#9118=VECTOR ( 'NONE', #20479, 1000.000000000000000 ) ;
#9122=VERTEX_POINT ( 'NONE', #5649 ) ;
#9134=CARTESIAN_POINT ( 'NONE',  ( 8.757878075398934925, -7.394122547431893011, -1.500000000000000000 ) ) ;
#9139=CIRCLE ( 'NONE', #23568, 0.6002263538043648428 ) ;
#9160=CARTESIAN_POINT ( 'NONE',  ( 9.301547456646380496, 8.591538895647095941, -1.500000000000000000 ) ) ;
#9173=ORIENTED_EDGE ( 'NONE', *, *, #2724, .F. ) ;
#9177=CARTESIAN_POINT ( 'NONE',  ( 25.10445388623454477, -25.60065097860747585, 1.500000000000000000 ) ) ;
#9188=CARTESIAN_POINT ( 'NONE',  ( -4.163336342344337027E-14, 1.387778780781445676E-14, -1.500000000000000000 ) ) ;
#9197=DIRECTION ( 'NONE',  ( 1.000000000000000000, 0.000000000000000000, 0.000000000000000000 ) ) ;
#9200=ORIENTED_EDGE ( 'NONE', *, *, #9245, .T. ) ;
#9222=CARTESIAN_POINT ( 'NONE',  ( 3.221450758838616757, -1.621276839356792454, 1.500000000000000000 ) ) ;
#9223=ORIENTED_EDGE ( 'NONE', *, *, #22532, .F. ) ;
#9228=CIRCLE ( 'NONE', #10227, 0.6002263538043630664 ) ;
#9232=DIRECTION ( 'NONE',  ( -0.000000000000000000, 0.000000000000000000, 1.000000000000000000 ) ) ;
#9236=ORIENTED_EDGE ( 'NONE', *, *, #11998, .T. ) ;
#9245=EDGE_CURVE ( 'NONE', #24522, #27352, #15611, .T. ) ;
#9256=VECTOR ( 'NONE', #30244, 1000.000000000000000 ) ;
#9303=LINE ( 'NONE', #13546, #4859 ) ;
#9306=( BOUNDED_CURVE ( )  B_SPLINE_CURVE ( 3, ( #15060, #3689, #1041, #27234 ),
 .UNSPECIFIED., .F., .T. ) 
 B_SPLINE_CURVE_WITH_KNOTS ( ( 4, 4 ),
 ( 0.8137667884748612801, 2.327825865114931947 ),
 .UNSPECIFIED. ) 
 CURVE ( )  GEOMETRIC_REPRESENTATION_ITEM ( )  RATIONAL_B_SPLINE_CURVE ( ( 1.000000000000000000, 0.8179194830933627092, 0.8179194830933627092, 1.000000000000000000 ) ) 
 REPRESENTATION_ITEM ( '' )  );
#9307=LINE ( 'NONE', #2601, #11333 ) ;
#9315=DIRECTION ( 'NONE',  ( 0.4495526574063634095, -0.8932538319083086487, 0.000000000000000000 ) ) ;
#9327=ADVANCED_FACE ( 'NONE', ( #10955 ), #11099, .F. ) ;
#9332=CIRCLE ( 'NONE', #26272, 28.20443790117963800 ) ;
#9341=AXIS2_PLACEMENT_3D ( 'NONE', #6128, #18298, #8944 ) ;
#9342=VERTEX_POINT ( 'NONE', #4987 ) ;
#9357=AXIS2_PLACEMENT_3D ( 'NONE', #17246, #22070, #864 ) ;
#9375=ADVANCED_FACE ( 'NONE', ( #23686 ), #6863, .T. ) ;
#9384=AXIS2_PLACEMENT_3D ( 'NONE', #20361, #6010, #3677 ) ;
#9405=VERTEX_POINT ( 'NONE', #11701 ) ;
#9407=DIRECTION ( 'NONE',  ( 1.000000000000000000, 0.000000000000000000, 0.000000000000000000 ) ) ;
#9424=ORIENTED_EDGE ( 'NONE', *, *, #27118, .F. ) ;
#9427=VERTEX_POINT ( 'NONE', #12637 ) ;
#9430=EDGE_CURVE ( 'NONE', #5262, #10442, #8357, .T. ) ;
#9435=ORIENTED_EDGE ( 'NONE', *, *, #27469, .F. ) ;
#9438=CARTESIAN_POINT ( 'NONE',  ( 26.36764545593177544, -31.31467416275353344, 1.500000000000000000 ) ) ;
#9441=AXIS2_PLACEMENT_3D ( 'NONE', #9188, #18248, #28208 ) ;
#9456=ORIENTED_EDGE ( 'NONE', *, *, #22321, .F. ) ;
#9466=ORIENTED_EDGE ( 'NONE', *, *, #14365, .F. ) ;
#9469=CARTESIAN_POINT ( 'NONE',  ( 24.03057240117691862, 26.57182937991349903, 1.500000000000000000 ) ) ;
#9475=AXIS2_PLACEMENT_3D ( 'NONE', #24519, #12689, #29844 ) ;
#9477=DIRECTION ( 'NONE',  ( -0.000000000000000000, 0.000000000000000000, 1.000000000000000000 ) ) ;
#9486=CARTESIAN_POINT ( 'NONE',  ( 0.000000000000000000, 0.000000000000000000, 0.000000000000000000 ) ) ;
#9489=CARTESIAN_POINT ( 'NONE',  ( -4.163336342344337027E-14, -1.387778780781445676E-14, -1.500000000000000000 ) ) ;
#9499=LINE ( 'NONE', #23381, #5114 ) ;
#9511=ORIENTED_EDGE ( 'NONE', *, *, #10956, .T. ) ;
#9517=DIRECTION ( 'NONE',  ( 0.000000000000000000, -0.000000000000000000, -1.000000000000000000 ) ) ;
#9518=CARTESIAN_POINT ( 'NONE',  ( 28.37932450449293853, 10.51822134874671022, -1.500000000000000000 ) ) ;
#9522=CARTESIAN_POINT ( 'NONE',  ( 8.860628911697515875, 8.184276679720483116, 1.500000000000000000 ) ) ;
#9526=ORIENTED_EDGE ( 'NONE', *, *, #3733, .F. ) ;
#9538=CARTESIAN_POINT ( 'NONE',  ( 17.22181377297005866, 14.41708049311048789, -1.500000000000000000 ) ) ;
#9556=CARTESIAN_POINT ( 'NONE',  ( -17.84153987719600920, 14.83584055149731284, -1.500000000000000000 ) ) ;
#9558=DIRECTION ( 'NONE',  ( -0.000000000000000000, 0.000000000000000000, 1.000000000000000000 ) ) ;
#9571=ADVANCED_FACE ( 'NONE', ( #24624 ), #468, .F. ) ;
#9577=CIRCLE ( 'NONE', #9034, 2.898871837527149609 ) ;
#9594=AXIS2_PLACEMENT_3D ( 'NONE', #17575, #8072, #5716 ) ;
#9597=DIRECTION ( 'NONE',  ( -0.6707505147970090897, -0.7416830501633074890, 0.000000000000000000 ) ) ;
#9612=EDGE_CURVE ( 'NONE', #7103, #479, #10323, .T. ) ;
#9627=CARTESIAN_POINT ( 'NONE',  ( 22.95669091611928181, 27.54300778121952575, -1.500000000000000000 ) ) ;
#9662=DIRECTION ( 'NONE',  ( 0.4495526574063634095, 0.8932538319083086487, 0.000000000000000000 ) ) ;
#9668=DIRECTION ( 'NONE',  ( -0.000000000000000000, -0.000000000000000000, -1.000000000000000000 ) ) ;
#9675=ORIENTED_EDGE ( 'NONE', *, *, #8275, .T. ) ;
#9684=ORIENTED_EDGE ( 'NONE', *, *, #20469, .T. ) ;
#9686=DIRECTION ( 'NONE',  ( 1.000000000000000000, 0.000000000000000000, 0.000000000000000000 ) ) ;
#9694=CARTESIAN_POINT ( 'NONE',  ( 19.54426622602689179, 37.07991288358296345, -1.499999999999999778 ) ) ;
#9709=CARTESIAN_POINT ( 'NONE',  ( 14.41708049311143469, -17.22181377297010130, 1.500000000000000000 ) ) ;
#9717=ORIENTED_EDGE ( 'NONE', *, *, #16616, .T. ) ;
#9726=CARTESIAN_POINT ( 'NONE',  ( -15.57266529552203416, -38.96488032230103471, -1.500000000000000000 ) ) ;
#9738=EDGE_CURVE ( 'NONE', #7027, #16799, #15823, .T. ) ;
#9746=ADVANCED_FACE ( 'NONE', ( #8364 ), #12432, .F. ) ;
#9748=ORIENTED_EDGE ( 'NONE', *, *, #17781, .F. ) ;
#9757=EDGE_CURVE ( 'NONE', #21725, #25705, #5702, .T. ) ;
#9765=AXIS2_PLACEMENT_3D ( 'NONE', #13595, #1272, #3607 ) ;
#9768=DIRECTION ( 'NONE',  ( 0.6707505147970127535, 0.7416830501633041584, 0.000000000000000000 ) ) ;
#9776=AXIS2_PLACEMENT_3D ( 'NONE', #19838, #12984, #1122 ) ;
#9786=AXIS2_PLACEMENT_3D ( 'NONE', #11054, #8572, #15414 ) ;
#9799=AXIS2_PLACEMENT_3D ( 'NONE', #29232, #3337, #12869 ) ;
#9801=ORIENTED_EDGE ( 'NONE', *, *, #6854, .F. ) ;
#9807=ADVANCED_FACE ( 'NONE', ( #22994 ), #27994, .F. ) ;
#9813=DIRECTION ( 'NONE',  ( -0.000000000000000000, 0.000000000000000000, 1.000000000000000000 ) ) ;
#9829=AXIS2_PLACEMENT_3D ( 'NONE', #9222, #18737, #28251 ) ;
#9862=CARTESIAN_POINT ( 'NONE',  ( -6.414842543015754295, 17.06554576617236307, 1.500000000000000000 ) ) ;
#9871=AXIS2_PLACEMENT_3D ( 'NONE', #20127, #12962, #27154 ) ;
#9891=CARTESIAN_POINT ( 'NONE',  ( -22.95669091611927826, -27.54300778121952220, 1.500000000000000000 ) ) ;
#9894=CIRCLE ( 'NONE', #4416, 14.52510309069108807 ) ;
#9903=ORIENTED_EDGE ( 'NONE', *, *, #12895, .T. ) ;
#9911=AXIS2_PLACEMENT_3D ( 'NONE', #19414, #19249, #5796 ) ;
#9920=VERTEX_POINT ( 'NONE', #7229 ) ;
#9922=EDGE_CURVE ( 'NONE', #7456, #17335, #13519, .T. ) ;
#9927=VERTEX_POINT ( 'NONE', #29222 ) ;
#9954=ORIENTED_EDGE ( 'NONE', *, *, #16616, .F. ) ;
#9956=FACE_OUTER_BOUND ( 'NONE', #722, .T. ) ;
#9960=EDGE_CURVE ( 'NONE', #14341, #7065, #19802, .T. ) ;
#9991=EDGE_CURVE ( 'NONE', #10311, #9122, #7298, .T. ) ;
#9992=ORIENTED_EDGE ( 'NONE', *, *, #192, .T. ) ;
#9994=DIRECTION ( 'NONE',  ( -0.000000000000000000, -0.000000000000000000, -1.000000000000000000 ) ) ;
#10006=CARTESIAN_POINT ( 'NONE',  ( 1.073881485057758711, -0.9711784013061475207, 1.500000000000000000 ) ) ;
#10013=ORIENTED_EDGE ( 'NONE', *, *, #25981, .F. ) ;
#10029=VECTOR ( 'NONE', #10908, 1000.000000000000114 ) ;
#10033=FACE_OUTER_BOUND ( 'NONE', #29993, .T. ) ;
#10050=AXIS2_PLACEMENT_3D ( 'NONE', #4141, #16303, #18501 ) ;
#10097=DIRECTION ( 'NONE',  ( -0.000000000000000000, -0.000000000000000000, -1.000000000000000000 ) ) ;
#10104=ORIENTED_EDGE ( 'NONE', *, *, #25557, .T. ) ;
#10149=DIRECTION ( 'NONE',  ( -0.000000000000000000, 0.000000000000000000, 1.000000000000000000 ) ) ;
#10158=AXIS2_PLACEMENT_3D ( 'NONE', #4244, #10821, #23112 ) ;
#10166=CARTESIAN_POINT ( 'NONE',  ( -25.10445388623454477, 25.60065097860747585, 1.500000000000000000 ) ) ;
#10179=ORIENTED_EDGE ( 'NONE', *, *, #11860, .F. ) ;
#10185=DIRECTION ( 'NONE',  ( 1.000000000000000000, 0.000000000000000000, 0.000000000000000000 ) ) ;
#10186=AXIS2_PLACEMENT_3D ( 'NONE', #15258, #29482, #24629 ) ;
#10190=DIRECTION ( 'NONE',  ( -0.000000000000000000, 0.000000000000000000, 1.000000000000000000 ) ) ;
#10191=VERTEX_POINT ( 'NONE', #22576 ) ;
#10196=ORIENTED_EDGE ( 'NONE', *, *, #17435, .T. ) ;
#10227=AXIS2_PLACEMENT_3D ( 'NONE', #12991, #17985, #29986 ) ;
#10231=CARTESIAN_POINT ( 'NONE',  ( 0.000000000000000000, 0.000000000000000000, -1.500000000000000000 ) ) ;
#10233=CARTESIAN_POINT ( 'NONE',  ( 26.36764545593177544, -31.31467416275353344, -1.500000000000000000 ) ) ;
#10247=ORIENTED_EDGE ( 'NONE', *, *, #17534, .T. ) ;
#10262=CARTESIAN_POINT ( 'NONE',  ( -26.36764545593177900, 31.31467416275353344, 1.500000000000000000 ) ) ;
#10274=CARTESIAN_POINT ( 'NONE',  ( 9.216505592218814158, -7.781333699927420966, 1.500000000000000000 ) ) ;
#10279=CARTESIAN_POINT ( 'NONE',  ( 43.34097750826428097, 11.89502811014149763, 1.500000000000000444 ) ) ;
#10280=LINE ( 'NONE', #15111, #18360 ) ;
#10298=DIRECTION ( 'NONE',  ( -0.000000000000000000, -0.000000000000000000, -1.000000000000000000 ) ) ;
#10311=VERTEX_POINT ( 'NONE', #2453 ) ;
#10321=DIRECTION ( 'NONE',  ( -1.000000000000000000, 0.000000000000000000, 0.000000000000000000 ) ) ;
#10323=CIRCLE ( 'NONE', #22271, 12.66227964008302287 ) ;
#10333=CARTESIAN_POINT ( 'NONE',  ( 26.31795596221988376, 10.51822134874671022, 1.500000000000000000 ) ) ;
#10337=FACE_OUTER_BOUND ( 'NONE', #28602, .T. ) ;
#10338=EDGE_LOOP ( 'NONE', ( #26731, #3758, #23380, #12548, #28552 ) ) ;
#10341=DIRECTION ( 'NONE',  ( -0.000000000000000000, 0.000000000000000000, 1.000000000000000000 ) ) ;
#10349=CARTESIAN_POINT ( 'NONE',  ( -14.41708049311053053, 17.22181377296911720, -1.500000000000000000 ) ) ;
#10354=CARTESIAN_POINT ( 'NONE',  ( 26.36764545593177544, -31.31467416275353344, 1.500000000000000000 ) ) ;
#10368=AXIS2_PLACEMENT_3D ( 'NONE', #17556, #27074, #15194 ) ;
#10371=AXIS2_PLACEMENT_3D ( 'NONE', #23107, #13479, #6127 ) ;
#10385=EDGE_CURVE ( 'NONE', #3354, #16254, #22688, .T. ) ;
#10387=ORIENTED_EDGE ( 'NONE', *, *, #26720, .F. ) ;
#10400=CARTESIAN_POINT ( 'NONE',  ( 3.637110358602582583, 19.99473753024312117, -1.500000000000000000 ) ) ;
#10414=DIRECTION ( 'NONE',  ( -0.000000000000000000, 0.000000000000000000, 1.000000000000000000 ) ) ;
#10421=VERTEX_POINT ( 'NONE', #876 ) ;
#10423=ORIENTED_EDGE ( 'NONE', *, *, #16806, .F. ) ;
#10433=FACE_OUTER_BOUND ( 'NONE', #20773, .T. ) ;
#10442=VERTEX_POINT ( 'NONE', #12902 ) ;
#10447=ORIENTED_EDGE ( 'NONE', *, *, #25245, .F. ) ;
#10450=DIRECTION ( 'NONE',  ( -1.000000000000000000, 0.000000000000000000, 0.000000000000000000 ) ) ;
#10453=CIRCLE ( 'NONE', #17428, 32.32717498572574755 ) ;
#10465=DIRECTION ( 'NONE',  ( 0.000000000000000000, -0.000000000000000000, -1.000000000000000000 ) ) ;
#10482=DIRECTION ( 'NONE',  ( 1.000000000000000000, 0.000000000000000000, 0.000000000000000000 ) ) ;
#10493=ORIENTED_EDGE ( 'NONE', *, *, #19324, .T. ) ;
#10494=DIRECTION ( 'NONE',  ( -0.000000000000000000, 0.000000000000000000, 1.000000000000000000 ) ) ;
#10495=ADVANCED_FACE ( 'NONE', ( #20368 ), #27232, .F. ) ;
#10501=DIRECTION ( 'NONE',  ( 1.000000000000000000, 0.000000000000000000, 0.000000000000000000 ) ) ;
#10505=ADVANCED_FACE ( 'NONE', ( #3371 ), #15367, .F. ) ;
#10509=DIRECTION ( 'NONE',  ( -1.000000000000000000, 0.000000000000000000, 0.000000000000000000 ) ) ;
#10536=EDGE_CURVE ( 'NONE', #22024, #15589, #27223, .T. ) ;
#10537=DIRECTION ( 'NONE',  ( -0.000000000000000000, -0.000000000000000000, -1.000000000000000000 ) ) ;
#10538=EDGE_CURVE ( 'NONE', #21725, #15101, #15778, .T. ) ;
#10546=DIRECTION ( 'NONE',  ( -1.000000000000000000, 0.000000000000000000, 0.000000000000000000 ) ) ;
#10548=DIRECTION ( 'NONE',  ( -1.000000000000000000, 0.000000000000000000, 0.000000000000000000 ) ) ;
#10549=DIRECTION ( 'NONE',  ( 1.000000000000000000, 0.000000000000000000, 0.000000000000000000 ) ) ;
#10550=CARTESIAN_POINT ( 'NONE',  ( 17.22181377297005866, 14.41708049311048789, 1.500000000000000000 ) ) ;
#10561=EDGE_CURVE ( 'NONE', #479, #30031, #24226, .T. ) ;
#10562=DIRECTION ( 'NONE',  ( 0.000000000000000000, -0.000000000000000000, -1.000000000000000000 ) ) ;
#10572=FACE_OUTER_BOUND ( 'NONE', #12270, .T. ) ;
#10583=CARTESIAN_POINT ( 'NONE',  ( -12.66227964008306550, -1.387778780781445676E-14, 1.500000000000000000 ) ) ;
#10629=DIRECTION ( 'NONE',  ( 1.000000000000000000, 0.000000000000000000, 0.000000000000000000 ) ) ;
#10630=VERTEX_POINT ( 'NONE', #25189 ) ;
#10636=CIRCLE ( 'NONE', #1176, 0.6002263538043630664 ) ;
#10638=LINE ( 'NONE', #20149, #30326 ) ;
#10666=ADVANCED_FACE ( 'NONE', ( #25515 ), #18644, .F. ) ;
#10668=CARTESIAN_POINT ( 'NONE',  ( -15.57266529552203416, 38.96488032230103471, 1.500000000000000000 ) ) ;
#10686=CARTESIAN_POINT ( 'NONE',  ( -4.163336342344337027E-14, -1.387778780781445676E-14, 1.500000000000000000 ) ) ;
#10687=EDGE_CURVE ( 'NONE', #15112, #5146, #21110, .T. ) ;
#10696=CARTESIAN_POINT ( 'NONE',  ( -4.163336342344337027E-14, -1.387778780781445676E-14, 1.500000000000000000 ) ) ;
#10699=AXIS2_PLACEMENT_3D ( 'NONE', #10714, #29744, #28015 ) ;
#10702=ORIENTED_EDGE ( 'NONE', *, *, #30696, .F. ) ;
#10703=EDGE_CURVE ( 'NONE', #479, #20644, #1505, .T. ) ;
#10712=DIRECTION ( 'NONE',  ( -0.000000000000000000, -0.000000000000000000, -1.000000000000000000 ) ) ;
#10713=ADVANCED_FACE ( 'NONE', ( #14378 ), #11323, .F. ) ;
#10714=CARTESIAN_POINT ( 'NONE',  ( -24.03057240117691862, 26.57182937991349903, -1.500000000000000000 ) ) ;
#10715=EDGE_CURVE ( 'NONE', #11332, #5262, #18282, .T. ) ;
#10717=EDGE_LOOP ( 'NONE', ( #13248, #12341, #25264, #16057 ) ) ;
#10727=ORIENTED_EDGE ( 'NONE', *, *, #1172, .F. ) ;
#10734=VECTOR ( 'NONE', #21929, 1000.000000000000000 ) ;
#10737=CARTESIAN_POINT ( 'NONE',  ( 13.93942108199810193, -16.65122935894600076, -1.500000000000000000 ) ) ;
#10757=ORIENTED_EDGE ( 'NONE', *, *, #6548, .F. ) ;
#10770=ORIENTED_EDGE ( 'NONE', *, *, #29594, .F. ) ;
#10773=LINE ( 'NONE', #22768, #7610 ) ;
#10789=CYLINDRICAL_SURFACE ( 'NONE', #16115, 0.7441270634456903510 ) ;
#10797=VECTOR ( 'NONE', #25357, 1000.000000000000000 ) ;
#10798=AXIS2_PLACEMENT_3D ( 'NONE', #29395, #7876, #17685 ) ;
#10802=CYLINDRICAL_SURFACE ( 'NONE', #9475, 1.447898107987198646 ) ;
#10805=DIRECTION ( 'NONE',  ( -0.000000000000000000, -0.000000000000000000, -1.000000000000000000 ) ) ;
#10808=AXIS2_PLACEMENT_3D ( 'NONE', #30304, #8780, #22968 ) ;
#10821=DIRECTION ( 'NONE',  ( -0.000000000000000000, -0.000000000000000000, -1.000000000000000000 ) ) ;
#10830=AXIS2_PLACEMENT_3D ( 'NONE', #9538, #11578, #21220 ) ;
#10831=DIRECTION ( 'NONE',  ( 1.000000000000000000, 0.000000000000000000, 0.000000000000000000 ) ) ;
#10832=CIRCLE ( 'NONE', #11348, 2.898871837527151385 ) ;
#10842=VECTOR ( 'NONE', #2949, 1000.000000000000000 ) ;
#10867=DIRECTION ( 'NONE',  ( -0.000000000000000000, -0.000000000000000000, -1.000000000000000000 ) ) ;
#10879=ORIENTED_EDGE ( 'NONE', *, *, #6155, .F. ) ;
#10883=AXIS2_PLACEMENT_3D ( 'NONE', #821, #29215, #27190 ) ;
#10896=ADVANCED_FACE ( 'NONE', ( #494 ), #7992, .F. ) ;
#10908=DIRECTION ( 'NONE',  ( -0.6707505147970090897, 0.7416830501633074890, 0.000000000000000000 ) ) ;
#10909=FACE_BOUND ( 'NONE', #13354, .T. ) ;
#10938=ORIENTED_EDGE ( 'NONE', *, *, #17585, .F. ) ;
#10942=DIRECTION ( 'NONE',  ( -0.000000000000000000, -0.000000000000000000, -1.000000000000000000 ) ) ;
#10945=CIRCLE ( 'NONE', #27393, 12.66227964008308682 ) ;
#10955=FACE_OUTER_BOUND ( 'NONE', #19280, .T. ) ;
#10956=EDGE_CURVE ( 'NONE', #21029, #27347, #3788, .T. ) ;
#10977=CARTESIAN_POINT ( 'NONE',  ( 16.47768670952434178, 14.41708049311048789, -1.500000000000000000 ) ) ;
#10978=AXIS2_PLACEMENT_3D ( 'NONE', #24163, #19187, #16698 ) ;
#10980=CARTESIAN_POINT ( 'NONE',  ( 24.03057240117691862, -26.57182937991349903, 1.500000000000000000 ) ) ;
#10988=EDGE_CURVE ( 'NONE', #16799, #10191, #28176, .T. ) ;
#11008=DIRECTION ( 'NONE',  ( 0.4495526574063634095, 0.8932538319083086487, 0.000000000000000000 ) ) ;
#11014=CARTESIAN_POINT ( 'NONE',  ( -12.66227964008306550, -1.387778780781445676E-14, 1.500000000000000000 ) ) ;
#11054=CARTESIAN_POINT ( 'NONE',  ( -14.36006998371493637, -17.26937953831884442, -1.500000000000000000 ) ) ;
#11055=VECTOR ( 'NONE', #28953, 1000.000000000000000 ) ;
#11057=ORIENTED_EDGE ( 'NONE', *, *, #1264, .T. ) ;
#11058=ORIENTED_EDGE ( 'NONE', *, *, #30067, .T. ) ;
#11069=VECTOR ( 'NONE', #23273, 1000.000000000000000 ) ;
#11081=FACE_OUTER_BOUND ( 'NONE', #14279, .T. ) ;
#11097=ORIENTED_EDGE ( 'NONE', *, *, #8203, .T. ) ;
#11099=CYLINDRICAL_SURFACE ( 'NONE', #21255, 2.061368542273053883 ) ;
#11105=CARTESIAN_POINT ( 'NONE',  ( 26.83043119477639138, -8.695877139419035728, -1.500000000000000000 ) ) ;
#11112=ADVANCED_FACE ( 'NONE', ( #29163 ), #26521, .F. ) ;
#11113=DIRECTION ( 'NONE',  ( 1.000000000000000000, 0.000000000000000000, 0.000000000000000000 ) ) ;
#11148=ORIENTED_EDGE ( 'NONE', *, *, #25245, .T. ) ;
#11154=AXIS2_PLACEMENT_3D ( 'NONE', #5368, #15171, #24537 ) ;
#11157=ORIENTED_EDGE ( 'NONE', *, *, #9757, .T. ) ;
#11161=EDGE_CURVE ( 'NONE', #7065, #22885, #22754, .T. ) ;
#11199=CARTESIAN_POINT ( 'NONE',  ( 17.22181377297005866, 14.41708049311048789, 1.500000000000000000 ) ) ;
#11202=FACE_BOUND ( 'NONE', #26647, .T. ) ;
#11242=DIRECTION ( 'NONE',  ( -1.000000000000000000, 0.000000000000000000, 0.000000000000000000 ) ) ;
#11243=CARTESIAN_POINT ( 'NONE',  ( 0.000000000000000000, 0.000000000000000000, 1.500000000000000000 ) ) ;
#11247=DIRECTION ( 'NONE',  ( -0.000000000000000000, -0.000000000000000000, -1.000000000000000000 ) ) ;
#11279=CARTESIAN_POINT ( 'NONE',  ( 26.73000961532937225, -9.331429872129930914, 1.500000000000000000 ) ) ;
#11288=CIRCLE ( 'NONE', #24227, 0.6002263538043630664 ) ;
#11299=CARTESIAN_POINT ( 'NONE',  ( 2.599508007902112006, 14.29059753516471964, 1.500000000000000000 ) ) ;
#11301=EDGE_CURVE ( 'NONE', #2551, #6787, #15119, .T. ) ;
#11323=( BOUNDED_SURFACE ( )  B_SPLINE_SURFACE ( 3, 1, ( 
 ( #16875, #19370 ),
 ( #30753, #11730 ),
 ( #28890, #9694 ),
 ( #23721, #2370 ) ),
 .UNSPECIFIED., .F., .F., .T. ) 
 B_SPLINE_SURFACE_WITH_KNOTS ( ( 4, 4 ),
 ( 2, 2 ),
 ( 0.000000000000000000, 1.000000000000000000 ),
 ( 0.000000000000000000, 1.000000000000000000 ),
 .UNSPECIFIED. ) 
 GEOMETRIC_REPRESENTATION_ITEM ( )  RATIONAL_B_SPLINE_SURFACE ( (
 ( 1.000000000000000000, 1.000000000000000000),
 ( 0.9908525036704132205, 0.9908525036704132205),
 ( 0.9908525036704132205, 0.9908525036704132205),
 ( 1.000000000000000000, 1.000000000000000000) ) ) 
 REPRESENTATION_ITEM ( '' )  SURFACE ( )  );
#11331=ORIENTED_EDGE ( 'NONE', *, *, #22687, .F. ) ;
#11332=VERTEX_POINT ( 'NONE', #23515 ) ;
#11333=VECTOR ( 'NONE', #9768, 1000.000000000000000 ) ;
#11348=AXIS2_PLACEMENT_3D ( 'NONE', #12277, #12591, #28961 ) ;
#11356=CARTESIAN_POINT ( 'NONE',  ( 9.999999999999959144, 1.510243460696181139E-14, 1.500000000000000000 ) ) ;
#11368=ORIENTED_EDGE ( 'NONE', *, *, #21194, .T. ) ;
#11374=ORIENTED_EDGE ( 'NONE', *, *, #21748, .T. ) ;
#11399=FACE_BOUND ( 'NONE', #20230, .T. ) ;
#11418=ORIENTED_EDGE ( 'NONE', *, *, #15070, .T. ) ;
#11435=LINE ( 'NONE', #27510, #2875 ) ;
#11458=DIRECTION ( 'NONE',  ( -0.000000000000000000, 0.000000000000000000, 1.000000000000000000 ) ) ;
#11469=ORIENTED_EDGE ( 'NONE', *, *, #28801, .T. ) ;
#11480=EDGE_CURVE ( 'NONE', #7845, #4361, #8136, .T. ) ;
#11490=ADVANCED_FACE ( 'NONE', ( #9956 ), #17120, .T. ) ;
#11512=FACE_OUTER_BOUND ( 'NONE', #15856, .T. ) ;
#11524=EDGE_LOOP ( 'NONE', ( #28294, #1059, #8355, #3087 ) ) ;
#11531=LINE ( 'NONE', #9177, #8706 ) ;
#11544=DIRECTION ( 'NONE',  ( 1.000000000000000000, -2.890115478905172036E-15, 0.000000000000000000 ) ) ;
#11547=CARTESIAN_POINT ( 'NONE',  ( -15.16120755655624741, 17.22181377296911720, 1.500000000000000000 ) ) ;
#11555=ORIENTED_EDGE ( 'NONE', *, *, #4774, .T. ) ;
#11563=VECTOR ( 'NONE', #23343, 1000.000000000000000 ) ;
#11565=CARTESIAN_POINT ( 'NONE',  ( -32.32717498572578307, -1.387778780781445676E-14, 1.500000000000000000 ) ) ;
#11567=ORIENTED_EDGE ( 'NONE', *, *, #25434, .T. ) ;
#11578=DIRECTION ( 'NONE',  ( -0.000000000000000000, 0.000000000000000000, 1.000000000000000000 ) ) ;
#11629=DIRECTION ( 'NONE',  ( 1.000000000000000000, 0.000000000000000000, 0.000000000000000000 ) ) ;
#11631=DIRECTION ( 'NONE',  ( -0.000000000000000000, -0.000000000000000000, -1.000000000000000000 ) ) ;
#11661=EDGE_CURVE ( 'NONE', #6974, #24290, #4795, .T. ) ;
#11666=ORIENTED_EDGE ( 'NONE', *, *, #7461, .F. ) ;
#11676=ORIENTED_EDGE ( 'NONE', *, *, #27685, .F. ) ;
#11679=ORIENTED_EDGE ( 'NONE', *, *, #25937, .F. ) ;
#11701=CARTESIAN_POINT ( 'NONE',  ( 30.75232512042845556, -9.966982604840845639, 1.500000000000000000 ) ) ;
#11717=DIRECTION ( 'NONE',  ( 1.000000000000000000, 0.000000000000000000, 0.000000000000000000 ) ) ;
#11727=DIRECTION ( 'NONE',  ( -0.000000000000000000, -0.000000000000000000, -1.000000000000000000 ) ) ;
#11730=CARTESIAN_POINT ( 'NONE',  ( 23.17581250239729940, 34.50630206824671120, -1.499999999999999778 ) ) ;
#11734=ORIENTED_EDGE ( 'NONE', *, *, #5236, .T. ) ;
#11751=EDGE_CURVE ( 'NONE', #15107, #15261, #11288, .T. ) ;
#11786=VECTOR ( 'NONE', #1046, 1000.000000000000000 ) ;
#11808=PLANE ( 'NONE',  #6052 ) ;
#11835=ORIENTED_EDGE ( 'NONE', *, *, #2713, .F. ) ;
#11856=ORIENTED_EDGE ( 'NONE', *, *, #16630, .T. ) ;
#11860=EDGE_CURVE ( 'NONE', #11332, #15421, #24198, .T. ) ;
#11866=DIRECTION ( 'NONE',  ( 1.000000000000000000, 0.000000000000000000, 0.000000000000000000 ) ) ;
#11875=AXIS2_PLACEMENT_3D ( 'NONE', #28269, #28422, #19201 ) ;
#11908=CARTESIAN_POINT ( 'NONE',  ( -15.10419704716067102, -17.26937953831884442, 1.500000000000000000 ) ) ;
#11917=AXIS2_PLACEMENT_3D ( 'NONE', #18016, #29551, #13333 ) ;
#11934=ORIENTED_EDGE ( 'NONE', *, *, #3260, .T. ) ;
#11941=ADVANCED_FACE ( 'NONE', ( #3951 ), #24678, .T. ) ;
#11946=CARTESIAN_POINT ( 'NONE',  ( -11.46182693247433804, -1.387778780781445676E-14, -1.500000000000000000 ) ) ;
#11967=CARTESIAN_POINT ( 'NONE',  ( -9.301547456646385825, 8.591538895647085283, 1.500000000000000000 ) ) ;
#11987=DIRECTION ( 'NONE',  ( -0.000000000000000000, -0.000000000000000000, -1.000000000000000000 ) ) ;
#11996=VERTEX_POINT ( 'NONE', #986 ) ;
#11998=EDGE_CURVE ( 'NONE', #20938, #3989, #15926, .T. ) ;
#12005=CARTESIAN_POINT ( 'NONE',  ( 0.000000000000000000, 0.000000000000000000, -1.500000000000000000 ) ) ;
#12014=EDGE_LOOP ( 'NONE', ( #5387, #9223, #5996, #16685 ) ) ;
#12015=CARTESIAN_POINT ( 'NONE',  ( -25.10445388623454477, -25.60065097860747585, 1.500000000000000000 ) ) ;
#12026=ORIENTED_EDGE ( 'NONE', *, *, #6962, .F. ) ;
#12065=CARTESIAN_POINT ( 'NONE',  ( -28.34828976096172681, -29.18752572968383063, 1.500000000000000000 ) ) ;
#12082=EDGE_CURVE ( 'NONE', #15261, #27429, #10945, .T. ) ;
#12094=VECTOR ( 'NONE', #17463, 1000.000000000000000 ) ;
#12101=DIRECTION ( 'NONE',  ( -0.000000000000000000, 0.000000000000000000, 1.000000000000000000 ) ) ;
#12111=ADVANCED_FACE ( 'NONE', ( #26680 ), #481, .F. ) ;
#12121=CARTESIAN_POINT ( 'NONE',  ( -8.757878075398936701, -7.394122547431892123, 1.500000000000000000 ) ) ;
#12125=DIRECTION ( 'NONE',  ( 1.000000000000000000, 0.000000000000000000, 0.000000000000000000 ) ) ;
#12127=CARTESIAN_POINT ( 'NONE',  ( 9.999999999999959144, 1.510243460696181139E-14, -1.500000000000000000 ) ) ;
#12133=ORIENTED_EDGE ( 'NONE', *, *, #19250, .T. ) ;
#12140=CARTESIAN_POINT ( 'NONE',  ( -13.93942108199721730, 16.65122935894503442, -1.500000000000000000 ) ) ;
#12147=DIRECTION ( 'NONE',  ( -1.000000000000000000, 0.000000000000000000, 0.000000000000000000 ) ) ;
#12150=CIRCLE ( 'NONE', #8688, 12.66227964008308682 ) ;
#12155=CARTESIAN_POINT ( 'NONE',  ( 14.36006998371584054, 17.26937953831785677, 1.500000000000000000 ) ) ;
#12163=ORIENTED_EDGE ( 'NONE', *, *, #29642, .F. ) ;
#12189=CIRCLE ( 'NONE', #8212, 11.46182693247429718 ) ;
#12190=CARTESIAN_POINT ( 'NONE',  ( 0.000000000000000000, 5.590849009245238754, 1.500000000000000000 ) ) ;
#12199=CARTESIAN_POINT ( 'NONE',  ( -15.57266529552203416, -38.96488032230103471, 1.500000000000000000 ) ) ;
#12244=ADVANCED_FACE ( 'NONE', ( #3593 ), #25879, .T. ) ;
#12250=EDGE_CURVE ( 'NONE', #27956, #1725, #13444, .T. ) ;
#12254=DIRECTION ( 'NONE',  ( 0.4495526574063634095, 0.8932538319083086487, 0.000000000000000000 ) ) ;
#12257=EDGE_CURVE ( 'NONE', #6050, #21077, #13928, .T. ) ;
#12267=CARTESIAN_POINT ( 'NONE',  ( -22.95669091611927826, 27.54300778121952220, 1.500000000000000000 ) ) ;
#12270=EDGE_LOOP ( 'NONE', ( #21986, #11157, #20871, #1833 ) ) ;
#12277=CARTESIAN_POINT ( 'NONE',  ( 3.118309183252346628, -17.14266753270391774, 1.500000000000000000 ) ) ;
#12283=CARTESIAN_POINT ( 'NONE',  ( -1.073881485057738949, -0.9711784013061123266, 1.500000000000000000 ) ) ;
#12286=AXIS2_PLACEMENT_3D ( 'NONE', #3139, #10149, #9686 ) ;
#12291=AXIS2_PLACEMENT_3D ( 'NONE', #16967, #7306, #26486 ) ;
#12300=LINE ( 'NONE', #14478, #10842 ) ;
#12317=EDGE_CURVE ( 'NONE', #8309, #25705, #20393, .T. ) ;
#12321=VERTEX_POINT ( 'NONE', #6547 ) ;
#12325=CARTESIAN_POINT ( 'NONE',  ( 28.34828976096171971, 29.18752572968384129, 1.500000000000000000 ) ) ;
#12338=CYLINDRICAL_SURFACE ( 'NONE', #10978, 11.46182693247435935 ) ;
#12341=ORIENTED_EDGE ( 'NONE', *, *, #17186, .T. ) ;
#12354=CARTESIAN_POINT ( 'NONE',  ( -26.36764545593178255, -31.31467416275353344, -1.500000000000000000 ) ) ;
#12374=ORIENTED_EDGE ( 'NONE', *, *, #25434, .F. ) ;
#12408=VERTEX_POINT ( 'NONE', #17578 ) ;
#12412=DIRECTION ( 'NONE',  ( 1.000000000000000000, 0.000000000000000000, 0.000000000000000000 ) ) ;
#12432=CYLINDRICAL_SURFACE ( 'NONE', #6293, 10.00000000000000000 ) ;
#12433=EDGE_LOOP ( 'NONE', ( #28910, #927, #29209, #26085 ) ) ;
#12437=LINE ( 'NONE', #7593, #10734 ) ;
#12447=DIRECTION ( 'NONE',  ( -0.000000000000000000, -0.000000000000000000, -1.000000000000000000 ) ) ;
#12448=VECTOR ( 'NONE', #10097, 1000.000000000000000 ) ;
#12451=ORIENTED_EDGE ( 'NONE', *, *, #5172, .F. ) ;
#12484=ORIENTED_EDGE ( 'NONE', *, *, #5236, .F. ) ;
#12487=CARTESIAN_POINT ( 'NONE',  ( 43.34097750826426676, -11.89502811014148698, 1.500000000000000444 ) ) ;
#12501=CARTESIAN_POINT ( 'NONE',  ( 8.860628911697515875, 8.184276679720483116, 1.500000000000000000 ) ) ;
#12508=CARTESIAN_POINT ( 'NONE',  ( -4.163336342344337027E-14, -1.387778780781445676E-14, -1.500000000000000000 ) ) ;
#12516=VERTEX_POINT ( 'NONE', #17722 ) ;
#12527=DIRECTION ( 'NONE',  ( 0.000000000000000000, -0.000000000000000000, -1.000000000000000000 ) ) ;
#12529=VECTOR ( 'NONE', #25471, 1000.000000000000000 ) ;
#12533=CARTESIAN_POINT ( 'NONE',  ( 0.000000000000000000, 0.000000000000000000, 1.500000000000000000 ) ) ;
#12534=CARTESIAN_POINT ( 'NONE',  ( -43.34097750826426676, 11.89502811014148698, -1.500000000000000444 ) ) ;
#12547=CARTESIAN_POINT ( 'NONE',  ( -15.57266529552203416, -38.96488032230103471, 1.500000000000000000 ) ) ;
#12548=ORIENTED_EDGE ( 'NONE', *, *, #22496, .F. ) ;
#12558=CARTESIAN_POINT ( 'NONE',  ( -15.57266529552203416, -38.96488032230103471, -1.500000000000000000 ) ) ;
#12562=DIRECTION ( 'NONE',  ( -0.000000000000000000, -0.000000000000000000, -1.000000000000000000 ) ) ;
#12573=LINE ( 'NONE', #701, #4832 ) ;
#12575=AXIS2_PLACEMENT_3D ( 'NONE', #5160, #3719, #320 ) ;
#12579=CARTESIAN_POINT ( 'NONE',  ( -28.34828976096172681, -29.18752572968383419, -1.500000000000000000 ) ) ;
#12585=DIRECTION ( 'NONE',  ( -0.000000000000000000, -0.000000000000000000, -1.000000000000000000 ) ) ;
#12591=DIRECTION ( 'NONE',  ( 0.000000000000000000, -0.000000000000000000, -1.000000000000000000 ) ) ;
#12599=DIRECTION ( 'NONE',  ( -0.000000000000000000, 0.000000000000000000, 1.000000000000000000 ) ) ;
#12611=EDGE_CURVE ( 'NONE', #8309, #27352, #2985, .T. ) ;
#12614=DIRECTION ( 'NONE',  ( 1.000000000000000000, -2.396195514597832977E-15, 0.000000000000000000 ) ) ;
#12630=VERTEX_POINT ( 'NONE', #9134 ) ;
#12637=CARTESIAN_POINT ( 'NONE',  ( 28.34828976096172681, -29.18752572968383419, 1.500000000000000000 ) ) ;
#12652=ORIENTED_EDGE ( 'NONE', *, *, #7691, .F. ) ;
#12658=LINE ( 'NONE', #775, #27852 ) ;
#12666=CYLINDRICAL_SURFACE ( 'NONE', #19861, 1.447898107987198646 ) ;
#12667=CARTESIAN_POINT ( 'NONE',  ( -23.17581250239728519, -34.50630206824672541, -1.499999999999999778 ) ) ;
#12669=VERTEX_POINT ( 'NONE', #2108 ) ;
#12674=AXIS2_PLACEMENT_3D ( 'NONE', #15154, #27493, #15624 ) ;
#12683=DIRECTION ( 'NONE',  ( -0.000000000000000000, -0.000000000000000000, -1.000000000000000000 ) ) ;
#12689=DIRECTION ( 'NONE',  ( -0.000000000000000000, -0.000000000000000000, -1.000000000000000000 ) ) ;
#12699=CARTESIAN_POINT ( 'NONE',  ( -30.31220697679117393, 11.23460505553742550, -1.500000000000000000 ) ) ;
#12730=CYLINDRICAL_SURFACE ( 'NONE', #29293, 1.447898107987170890 ) ;
#12735=ORIENTED_EDGE ( 'NONE', *, *, #6915, .T. ) ;
#12740=DIRECTION ( 'NONE',  ( -0.000000000000000000, 0.000000000000000000, 1.000000000000000000 ) ) ;
#12745=FACE_OUTER_BOUND ( 'NONE', #6107, .T. ) ;
#12782=DIRECTION ( 'NONE',  ( -1.000000000000000000, 0.000000000000000000, 0.000000000000000000 ) ) ;
#12799=DIRECTION ( 'NONE',  ( 1.000000000000000000, 0.000000000000000000, 0.000000000000000000 ) ) ;
#12807=AXIS2_PLACEMENT_3D ( 'NONE', #14532, #21691, #18755 ) ;
#12808=DIRECTION ( 'NONE',  ( 0.6707505147970023174, 0.7416830501633134842, 0.000000000000000000 ) ) ;
#12810=ORIENTED_EDGE ( 'NONE', *, *, #5745, .T. ) ;
#12834=DIRECTION ( 'NONE',  ( -0.000000000000000000, 0.000000000000000000, 1.000000000000000000 ) ) ;
#12835=ADVANCED_FACE ( 'NONE', ( #388 ), #29087, .F. ) ;
#12869=DIRECTION ( 'NONE',  ( -1.000000000000000000, 0.000000000000000000, 0.000000000000000000 ) ) ;
#12876=CIRCLE ( 'NONE', #19824, 0.7441270634457337607 ) ;
#12889=LINE ( 'NONE', #26769, #889 ) ;
#12892=CARTESIAN_POINT ( 'NONE',  ( -28.20443790117967708, -1.387778780781445676E-14, 1.500000000000000000 ) ) ;
#12895=EDGE_CURVE ( 'NONE', #6285, #20644, #26355, .T. ) ;
#12901=CARTESIAN_POINT ( 'NONE',  ( -14.41708049311053053, 17.22181377296911720, 1.500000000000000000 ) ) ;
#12902=CARTESIAN_POINT ( 'NONE',  ( -16.65122935894506639, -13.93942108199812324, -1.500000000000000000 ) ) ;
#12909=VECTOR ( 'NONE', #19517, 1000.000000000000000 ) ;
#12916=LINE ( 'NONE', #29440, #15124 ) ;
#12929=CYLINDRICAL_SURFACE ( 'NONE', #20795, 21.71568325578193637 ) ;
#12931=CIRCLE ( 'NONE', #30350, 2.061368542273053883 ) ;
#12945=ORIENTED_EDGE ( 'NONE', *, *, #30388, .F. ) ;
#12953=CYLINDRICAL_SURFACE ( 'NONE', #15920, 12.66227964008308682 ) ;
#12960=ORIENTED_EDGE ( 'NONE', *, *, #26381, .F. ) ;
#12962=DIRECTION ( 'NONE',  ( -0.000000000000000000, 0.000000000000000000, 1.000000000000000000 ) ) ;
#12971=CARTESIAN_POINT ( 'NONE',  ( -15.57266529552202883, -38.96488032230103471, -1.500000000000000000 ) ) ;
#12984=DIRECTION ( 'NONE',  ( -0.000000000000000000, 0.000000000000000000, 1.000000000000000000 ) ) ;
#12991=CARTESIAN_POINT ( 'NONE',  ( 9.216505592218814158, -7.781333699927420966, -1.500000000000000000 ) ) ;
#12996=EDGE_CURVE ( 'NONE', #4388, #19078, #1460, .T. ) ;
#13002=EDGE_CURVE ( 'NONE', #27498, #4581, #13025, .T. ) ;
#13024=EDGE_LOOP ( 'NONE', ( #16779, #4525, #14551, #1049 ) ) ;
#13025=LINE ( 'NONE', #17541, #5945 ) ;
#13033=EDGE_CURVE ( 'NONE', #21717, #19170, #13910, .T. ) ;
#13050=CARTESIAN_POINT ( 'NONE',  ( 19.54426622602689179, 37.07991288358296345, -1.499999999999999778 ) ) ;
#13057=ORIENTED_EDGE ( 'NONE', *, *, #22730, .T. ) ;
#13060=CARTESIAN_POINT ( 'NONE',  ( 28.79137815760242702, -9.331429872129930914, 1.500000000000000000 ) ) ;
#13071=CARTESIAN_POINT ( 'NONE',  ( 16.47768670952434178, 14.41708049311048789, 1.500000000000000000 ) ) ;
#13080=DIRECTION ( 'NONE',  ( 0.000000000000000000, -0.000000000000000000, -1.000000000000000000 ) ) ;
#13091=DIRECTION ( 'NONE',  ( -0.000000000000000000, -0.000000000000000000, -1.000000000000000000 ) ) ;
#13100=CIRCLE ( 'NONE', #19563, 32.32717498572581860 ) ;
#13101=DIRECTION ( 'NONE',  ( -0.000000000000000000, -0.000000000000000000, -1.000000000000000000 ) ) ;
#13118=EDGE_LOOP ( 'NONE', ( #25070, #9435, #13584, #4801 ) ) ;
#13138=AXIS2_PLACEMENT_3D ( 'NONE', #14875, #8333, #10509 ) ;
#13143=AXIS2_PLACEMENT_3D ( 'NONE', #15582, #29630, #6071 ) ;
#13155=DIRECTION ( 'NONE',  ( -1.000000000000000000, 0.000000000000000000, 0.000000000000000000 ) ) ;
#13187=EDGE_CURVE ( 'NONE', #20644, #21650, #6501, .T. ) ;
#13197=CARTESIAN_POINT ( 'NONE',  ( 23.17581250239729940, 34.50630206824671831, -1.499999999999999778 ) ) ;
#13199=CARTESIAN_POINT ( 'NONE',  ( 0.000000000000000000, 0.000000000000000000, 1.500000000000000000 ) ) ;
#13205=ADVANCED_FACE ( 'NONE', ( #14848 ), #17036, .F. ) ;
#13244=CARTESIAN_POINT ( 'NONE',  ( 22.58267429318971864, 26.57182937991349903, -1.500000000000000000 ) ) ;
#13248=ORIENTED_EDGE ( 'NONE', *, *, #13033, .T. ) ;
#13253=VERTEX_POINT ( 'NONE', #14999 ) ;
#13254=CIRCLE ( 'NONE', #22683, 0.7441270634457181066 ) ;
#13276=ADVANCED_FACE ( 'NONE', ( #22633 ), #17823, .F. ) ;
#13287=CIRCLE ( 'NONE', #27732, 23.20393738267338790 ) ;
#13290=EDGE_LOOP ( 'NONE', ( #12652, #16659, #763, #19807 ) ) ;
#13329=CIRCLE ( 'NONE', #10830, 0.7441270634457181066 ) ;
#13331=AXIS2_PLACEMENT_3D ( 'NONE', #1275, #3461, #3295 ) ;
#13332=ORIENTED_EDGE ( 'NONE', *, *, #10715, .T. ) ;
#13333=DIRECTION ( 'NONE',  ( 1.000000000000000000, 0.000000000000000000, 0.000000000000000000 ) ) ;
#13354=EDGE_LOOP ( 'NONE', ( #25568, #14106 ) ) ;
#13379=CARTESIAN_POINT ( 'NONE',  ( -4.163336342344337027E-14, 1.387778780781445676E-14, -1.500000000000000000 ) ) ;
#13410=FACE_BOUND ( 'NONE', #17935, .T. ) ;
#13418=EDGE_CURVE ( 'NONE', #4932, #8309, #10638, .T. ) ;
#13432=DIRECTION ( 'NONE',  ( 0.6707505147970010961, -0.7416830501633147055, 0.000000000000000000 ) ) ;
#13444=CIRCLE ( 'NONE', #9441, 10.00000000000000000 ) ;
#13471=ORIENTED_EDGE ( 'NONE', *, *, #4019, .F. ) ;
#13479=DIRECTION ( 'NONE',  ( -0.000000000000000000, -0.000000000000000000, -1.000000000000000000 ) ) ;
#13491=ORIENTED_EDGE ( 'NONE', *, *, #3160, .T. ) ;
#13516=DIRECTION ( 'NONE',  ( -0.000000000000000000, -0.000000000000000000, -1.000000000000000000 ) ) ;
#13519=( BOUNDED_CURVE ( )  B_SPLINE_CURVE ( 3, ( #3493, #994, #3178, #12547 ),
 .UNSPECIFIED., .F., .T. ) 
 B_SPLINE_CURVE_WITH_KNOTS ( ( 4, 4 ),
 ( 2.399144907686414196, 2.730840413552699353 ),
 .UNSPECIFIED. ) 
 CURVE ( )  GEOMETRIC_REPRESENTATION_ITEM ( )  RATIONAL_B_SPLINE_CURVE ( ( 1.000000000000000000, 0.9908525036704132205, 0.9908525036704132205, 1.000000000000000000 ) ) 
 REPRESENTATION_ITEM ( '' )  );
#13520=DIRECTION ( 'NONE',  ( 1.000000000000000000, 0.000000000000000000, 0.000000000000000000 ) ) ;
#13542=EDGE_LOOP ( 'NONE', ( #18483, #24472, #17639, #19608 ) ) ;
#13545=CARTESIAN_POINT ( 'NONE',  ( -1.073881485057738949, 0.9711784013061123266, 1.500000000000000000 ) ) ;
#13546=CARTESIAN_POINT ( 'NONE',  ( 9.999999999999959144, 1.510243460696181139E-14, 1.500000000000000000 ) ) ;
#13563=EDGE_CURVE ( 'NONE', #26022, #22885, #27846, .T. ) ;
#13576=ORIENTED_EDGE ( 'NONE', *, *, #19285, .F. ) ;
#13578=ORIENTED_EDGE ( 'NONE', *, *, #6155, .T. ) ;
#13579=EDGE_CURVE ( 'NONE', #26950, #20068, #27252, .T. ) ;
#13584=ORIENTED_EDGE ( 'NONE', *, *, #15067, .T. ) ;
#13591=DIRECTION ( 'NONE',  ( -0.000000000000000000, 0.000000000000000000, 1.000000000000000000 ) ) ;
#13595=CARTESIAN_POINT ( 'NONE',  ( 0.000000000000000000, -5.590849009245238754, 1.500000000000000000 ) ) ;
#13603=CYLINDRICAL_SURFACE ( 'NONE', #28068, 21.71568325578132530 ) ;
#13604=EDGE_CURVE ( 'NONE', #1725, #27956, #21862, .T. ) ;
#13610=CARTESIAN_POINT ( 'NONE',  ( -6.414842543015754295, -17.06554576617236307, -1.500000000000000000 ) ) ;
#13624=UNCERTAINTY_MEASURE_WITH_UNIT (LENGTH_MEASURE( 1.000000000000000082E-05 ), #14769, 'distance_accuracy_value', 'NONE');
#13630=FACE_OUTER_BOUND ( 'NONE', #7261, .T. ) ;
#13657=ORIENTED_EDGE ( 'NONE', *, *, #4054, .T. ) ;
#13669=DIRECTION ( 'NONE',  ( -0.000000000000000000, -0.000000000000000000, -1.000000000000000000 ) ) ;
#13677=ORIENTED_EDGE ( 'NONE', *, *, #7277, .F. ) ;
#13686=ORIENTED_EDGE ( 'NONE', *, *, #26117, .T. ) ;
#13708=EDGE_LOOP ( 'NONE', ( #21936, #10702, #13057, #18023 ) ) ;
#13712=ORIENTED_EDGE ( 'NONE', *, *, #10538, .F. ) ;
#13718=ORIENTED_EDGE ( 'NONE', *, *, #20062, .F. ) ;
#13763=FACE_OUTER_BOUND ( 'NONE', #6112, .T. ) ;
#13764=DIRECTION ( 'NONE',  ( -0.000000000000000000, -0.000000000000000000, -1.000000000000000000 ) ) ;
#13766=AXIS2_PLACEMENT_3D ( 'NONE', #1073, #19947, #29464 ) ;
#13795=AXIS2_PLACEMENT_3D ( 'NONE', #2206, #28418, #19656 ) ;
#13797=ORIENTED_EDGE ( 'NONE', *, *, #22726, .F. ) ;
#13802=CIRCLE ( 'NONE', #22255, 0.7441270634457337607 ) ;
#13844=CARTESIAN_POINT ( 'NONE',  ( -1.073881485057887497, 0.9711784013062738641, -1.500000000000000000 ) ) ;
#13845=AXIS2_PLACEMENT_3D ( 'NONE', #6358, #30061, #18522 ) ;
#13870=CARTESIAN_POINT ( 'NONE',  ( 26.73000961532937225, -9.331429872129930914, -1.500000000000000000 ) ) ;
#13884=FACE_OUTER_BOUND ( 'NONE', #24959, .T. ) ;
#13885=ORIENTED_EDGE ( 'NONE', *, *, #8275, .F. ) ;
#13897=AXIS2_PLACEMENT_3D ( 'NONE', #13379, #1519, #1212 ) ;
#13900=VERTEX_POINT ( 'NONE', #8519 ) ;
#13910=CIRCLE ( 'NONE', #16894, 2.898871837527149609 ) ;
#13915=CARTESIAN_POINT ( 'NONE',  ( -4.100931858250860707, -19.90478481566557534, 1.500000000000000000 ) ) ;
#13928=CIRCLE ( 'NONE', #15413, 21.71568325578263625 ) ;
#13930=CARTESIAN_POINT ( 'NONE',  ( 3.221450758838616757, 1.621276839356792454, -1.500000000000000000 ) ) ;
#13943=EDGE_LOOP ( 'NONE', ( #3751, #24642, #734, #19336, #16730, #23708 ) ) ;
#13952=EDGE_CURVE ( 'NONE', #24522, #16767, #20086, .T. ) ;
#13956=DIRECTION ( 'NONE',  ( -0.000000000000000000, 0.000000000000000000, 1.000000000000000000 ) ) ;
#13957=CARTESIAN_POINT ( 'NONE',  ( 8.419710366748642372, 7.777014463793876509, 1.500000000000000000 ) ) ;
#13958=CARTESIAN_POINT ( 'NONE',  ( 15.57266529552201995, -38.96488032230103471, 1.500000000000000000 ) ) ;
#14023=DIRECTION ( 'NONE',  ( 1.000000000000000000, 0.000000000000000000, 0.000000000000000000 ) ) ;
#14027=FACE_BOUND ( 'NONE', #13943, .T. ) ;
#14044=DIRECTION ( 'NONE',  ( -0.6707505147970023174, -0.7416830501633134842, 0.000000000000000000 ) ) ;
#14045=ORIENTED_EDGE ( 'NONE', *, *, #29014, .T. ) ;
#14053=VECTOR ( 'NONE', #17263, 1000.000000000000000 ) ;
#14054=CARTESIAN_POINT ( 'NONE',  ( -13.93942108199721730, 16.65122935894503442, 1.500000000000000000 ) ) ;
#14062=ORIENTED_EDGE ( 'NONE', *, *, #3078, .T. ) ;
#14068=ORIENTED_EDGE ( 'NONE', *, *, #5034, .F. ) ;
#14079=LINE ( 'NONE', #11299, #29381 ) ;
#14106=ORIENTED_EDGE ( 'NONE', *, *, #18529, .F. ) ;
#14149=EDGE_CURVE ( 'NONE', #4573, #21077, #244, .T. ) ;
#14150=CARTESIAN_POINT ( 'NONE',  ( -25.10445388623454477, -25.60065097860747585, -1.500000000000000000 ) ) ;
#14154=FACE_OUTER_BOUND ( 'NONE', #20066, .T. ) ;
#14162=VERTEX_POINT ( 'NONE', #7216 ) ;
#14180=CIRCLE ( 'NONE', #28649, 0.6002263538043648428 ) ;
#14194=CARTESIAN_POINT ( 'NONE',  ( -12.66227964008306550, -1.387778780781445676E-14, -1.500000000000000000 ) ) ;
#14210=VECTOR ( 'NONE', #1651, 1000.000000000000000 ) ;
#14220=AXIS2_PLACEMENT_3D ( 'NONE', #19062, #28282, #16420 ) ;
#14224=ORIENTED_EDGE ( 'NONE', *, *, #3242, .T. ) ;
#14228=CARTESIAN_POINT ( 'NONE',  ( -43.34097750826428097, -11.89502811014147987, 1.500000000000000444 ) ) ;
#14229=ORIENTED_EDGE ( 'NONE', *, *, #7075, .F. ) ;
#14239=AXIS2_PLACEMENT_3D ( 'NONE', #1397, #25408, #29935 ) ;
#14254=ORIENTED_EDGE ( 'NONE', *, *, #26518, .T. ) ;
#14270=AXIS2_PLACEMENT_3D ( 'NONE', #26270, #4909, #19248 ) ;
#14279=EDGE_LOOP ( 'NONE', ( #26610, #2704, #9954, #11835 ) ) ;
#14286=AXIS2_PLACEMENT_3D ( 'NONE', #15280, #22457, #1106 ) ;
#14288=FACE_OUTER_BOUND ( 'NONE', #22664, .T. ) ;
#14299=AXIS2_PLACEMENT_3D ( 'NONE', #29962, #13591, #25587 ) ;
#14300=VERTEX_POINT ( 'NONE', #20315 ) ;
#14323=ADVANCED_FACE ( 'NONE', ( #22798 ), #18131, .F. ) ;
#14341=VERTEX_POINT ( 'NONE', #10333 ) ;
#14362=ADVANCED_FACE ( 'NONE', ( #25290 ), #10789, .F. ) ;
#14365=EDGE_CURVE ( 'NONE', #8763, #1352, #30119, .T. ) ;
#14375=CARTESIAN_POINT ( 'NONE',  ( 22.58267429318974706, -26.57182937991349903, 1.500000000000000000 ) ) ;
#14377=EDGE_LOOP ( 'NONE', ( #29140, #27427, #4969, #172 ) ) ;
#14378=FACE_OUTER_BOUND ( 'NONE', #22105, .T. ) ;
#14395=LINE ( 'NONE', #28439, #2125 ) ;
#14398=DIRECTION ( 'NONE',  ( 1.000000000000000000, 0.000000000000000000, 0.000000000000000000 ) ) ;
#14410=ORIENTED_EDGE ( 'NONE', *, *, #27534, .T. ) ;
#14436=DIRECTION ( 'NONE',  ( -1.000000000000000000, 0.000000000000000000, 0.000000000000000000 ) ) ;
#14437=ORIENTED_EDGE ( 'NONE', *, *, #5745, .F. ) ;
#14439=CIRCLE ( 'NONE', #7973, 11.46182693247429718 ) ;
#14453=CARTESIAN_POINT ( 'NONE',  ( 14.36006998371584054, 17.26937953831785677, 1.500000000000000000 ) ) ;
#14457=CARTESIAN_POINT ( 'NONE',  ( 0.000000000000000000, 0.000000000000000000, 1.500000000000000000 ) ) ;
#14478=CARTESIAN_POINT ( 'NONE',  ( 28.34828976096172681, 29.18752572968383419, 1.500000000000000000 ) ) ;
#14487=ADVANCED_FACE ( 'NONE', ( #4073 ), #13603, .T. ) ;
#14502=EDGE_CURVE ( 'NONE', #5698, #14945, #23687, .T. ) ;
#14532=CARTESIAN_POINT ( 'NONE',  ( 0.000000000000000000, 0.000000000000000000, -1.500000000000000000 ) ) ;
#14551=ORIENTED_EDGE ( 'NONE', *, *, #24795, .T. ) ;
#14563=ADVANCED_FACE ( 'NONE', ( #22285 ), #17690, .F. ) ;
#14574=CARTESIAN_POINT ( 'NONE',  ( 25.10445388623454477, 25.60065097860747585, -1.500000000000000000 ) ) ;
#14615=ORIENTED_EDGE ( 'NONE', *, *, #265, .T. ) ;
#14628=CARTESIAN_POINT ( 'NONE',  ( -28.34828976096172681, -29.18752572968383419, 1.500000000000000000 ) ) ;
#14669=VERTEX_POINT ( 'NONE', #3424 ) ;
#14689=DIRECTION ( 'NONE',  ( 1.000000000000000000, 0.000000000000000000, 0.000000000000000000 ) ) ;
#14692=EDGE_LOOP ( 'NONE', ( #11058, #629, #20195, #11934 ) ) ;
#14733=CIRCLE ( 'NONE', #22194, 0.7441270634457163302 ) ;
#14736=ORIENTED_EDGE ( 'NONE', *, *, #3490, .F. ) ;
#14737=EDGE_CURVE ( 'NONE', #20938, #4388, #5153, .T. ) ;
#14744=CIRCLE ( 'NONE', #288, 0.6002263538043648428 ) ;
#14749=DIRECTION ( 'NONE',  ( -0.000000000000000000, -0.000000000000000000, -1.000000000000000000 ) ) ;
#14758=CYLINDRICAL_SURFACE ( 'NONE', #14869, 0.7441270634457163302 ) ;
#14766=EDGE_CURVE ( 'NONE', #1105, #22982, #18405, .T. ) ;
#14768=AXIS2_PLACEMENT_3D ( 'NONE', #17420, #29894, #24897 ) ;
#14769=( LENGTH_UNIT ( ) NAMED_UNIT ( * ) SI_UNIT ( .MILLI., .METRE. ) );
#14793=CARTESIAN_POINT ( 'NONE',  ( 22.58267429318971864, 26.57182937991349903, 1.500000000000000000 ) ) ;
#14803=DIRECTION ( 'NONE',  ( -0.000000000000000000, -0.000000000000000000, -1.000000000000000000 ) ) ;
#14811=VECTOR ( 'NONE', #23177, 1000.000000000000000 ) ;
#14817=ORIENTED_EDGE ( 'NONE', *, *, #12250, .F. ) ;
#14824=CARTESIAN_POINT ( 'NONE',  ( -28.20443790117967708, -1.387778780781445676E-14, -1.500000000000000000 ) ) ;
#14826=VERTEX_POINT ( 'NONE', #1851 ) ;
#14834=LINE ( 'NONE', #24500, #19323 ) ;
#14848=FACE_OUTER_BOUND ( 'NONE', #29670, .T. ) ;
#14856=DIRECTION ( 'NONE',  ( -0.000000000000000000, -0.000000000000000000, -1.000000000000000000 ) ) ;
#14869=AXIS2_PLACEMENT_3D ( 'NONE', #21782, #717, #26313 ) ;
#14875=CARTESIAN_POINT ( 'NONE',  ( 17.22181377297005866, 14.41708049311048789, 1.500000000000000000 ) ) ;
#14885=LINE ( 'NONE', #22373, #16574 ) ;
#14910=AXIS2_PLACEMENT_3D ( 'NONE', #1707, #21026, #18700 ) ;
#14916=PRODUCT ( 'Front & Rear Ported Pressure', 'Front & Rear Ported Pressure', '', ( #26918 ) ) ;
#14919=DIRECTION ( 'NONE',  ( -0.000000000000000000, 0.000000000000000000, 1.000000000000000000 ) ) ;
#14945=VERTEX_POINT ( 'NONE', #14150 ) ;
#14951=CARTESIAN_POINT ( 'NONE',  ( -23.17581250239728519, 34.50630206824671831, 1.499999999999999778 ) ) ;
#14970=CARTESIAN_POINT ( 'NONE',  ( 22.58267429318971864, 26.57182937991349903, 1.500000000000000000 ) ) ;
#14979=DIRECTION ( 'NONE',  ( -1.000000000000000000, 0.000000000000000000, 0.000000000000000000 ) ) ;
#14980=AXIS2_PLACEMENT_3D ( 'NONE', #30142, #25000, #13155 ) ;
#14999=CARTESIAN_POINT ( 'NONE',  ( -21.71568325578193637, 0.000000000000000000, 1.500000000000000000 ) ) ;
#15001=CARTESIAN_POINT ( 'NONE',  ( -4.163336342344337027E-14, -1.387778780781445676E-14, 1.500000000000000000 ) ) ;
#15012=DIRECTION ( 'NONE',  ( 0.6707505147970023174, -0.7416830501633134842, 0.000000000000000000 ) ) ;
#15020=CARTESIAN_POINT ( 'NONE',  ( -3.221450758838616757, -1.621276839356792454, -1.500000000000000000 ) ) ;
#15046=DIRECTION ( 'NONE',  ( -0.6707505147970024284, -0.7416830501633134842, 0.000000000000000000 ) ) ;
#15054=CYLINDRICAL_SURFACE ( 'NONE', #20274, 14.52510309069108807 ) ;
#15060=CARTESIAN_POINT ( 'NONE',  ( -28.34828976096172681, 29.18752572968383419, -1.500000000000000000 ) ) ;
#15067=EDGE_CURVE ( 'NONE', #9122, #8016, #12150, .T. ) ;
#15070=EDGE_CURVE ( 'NONE', #20436, #19427, #17126, .T. ) ;
#15088=ORIENTED_EDGE ( 'NONE', *, *, #17241, .F. ) ;
#15090=EDGE_CURVE ( 'NONE', #3354, #7456, #12916, .T. ) ;
#15101=VERTEX_POINT ( 'NONE', #26476 ) ;
#15107=VERTEX_POINT ( 'NONE', #29126 ) ;
#15111=CARTESIAN_POINT ( 'NONE',  ( 22.95669091611932089, -27.54300778121948312, 1.500000000000000000 ) ) ;
#15112=VERTEX_POINT ( 'NONE', #28971 ) ;
#15119=LINE ( 'NONE', #15909, #9256 ) ;
#15120=DIRECTION ( 'NONE',  ( -0.6707505147970024284, 0.7416830501633134842, 0.000000000000000000 ) ) ;
#15123=CARTESIAN_POINT ( 'NONE',  ( 15.57266529552203416, 38.96488032230103471, 1.500000000000000000 ) ) ;
#15124=VECTOR ( 'NONE', #7457, 1000.000000000000114 ) ;
#15154=CARTESIAN_POINT ( 'NONE',  ( -14.36006998371493637, -17.26937953831884442, 1.500000000000000000 ) ) ;
#15171=DIRECTION ( 'NONE',  ( -0.000000000000000000, 0.000000000000000000, 1.000000000000000000 ) ) ;
#15194=DIRECTION ( 'NONE',  ( 1.000000000000000000, 0.000000000000000000, 0.000000000000000000 ) ) ;
#15196=CARTESIAN_POINT ( 'NONE',  ( -28.20443790117967708, -1.387778780781445676E-14, 1.500000000000000000 ) ) ;
#15225=DIRECTION ( 'NONE',  ( -1.000000000000000000, 0.000000000000000000, 0.000000000000000000 ) ) ;
#15227=DIRECTION ( 'NONE',  ( -1.000000000000000000, 0.000000000000000000, 0.000000000000000000 ) ) ;
#15229=CIRCLE ( 'NONE', #1809, 23.20393738267408779 ) ;
#15232=CIRCLE ( 'NONE', #9776, 23.20393738267338790 ) ;
#15238=VECTOR ( 'NONE', #18877, 1000.000000000000000 ) ;
#15244=AXIS2_PLACEMENT_3D ( 'NONE', #17675, #10190, #3026 ) ;
#15256=DIRECTION ( 'NONE',  ( -0.000000000000000000, -0.000000000000000000, -1.000000000000000000 ) ) ;
#15258=CARTESIAN_POINT ( 'NONE',  ( 28.79137815760242702, -9.331429872129930914, 1.500000000000000000 ) ) ;
#15261=VERTEX_POINT ( 'NONE', #19420 ) ;
#15269=CARTESIAN_POINT ( 'NONE',  ( -17.79239818699324616, -14.89473990422481187, -1.500000000000000000 ) ) ;
#15271=EDGE_CURVE ( 'NONE', #11996, #8846, #3195, .T. ) ;
#15280=CARTESIAN_POINT ( 'NONE',  ( -17.26937953831790651, 14.36006998371489551, 1.500000000000000000 ) ) ;
#15283=CYLINDRICAL_SURFACE ( 'NONE', #4323, 23.20393738267273420 ) ;
#15285=DIRECTION ( 'NONE',  ( -0.000000000000000000, -0.000000000000000000, -1.000000000000000000 ) ) ;
#15286=CARTESIAN_POINT ( 'NONE',  ( -15.57266529552202883, -38.96488032230103471, 1.500000000000000000 ) ) ;
#15294=ORIENTED_EDGE ( 'NONE', *, *, #2235, .F. ) ;
#15304=CARTESIAN_POINT ( 'NONE',  ( -4.163336342344337027E-14, 1.387778780781445676E-14, 1.500000000000000000 ) ) ;
#15352=ORIENTED_EDGE ( 'NONE', *, *, #25028, .F. ) ;
#15367=CYLINDRICAL_SURFACE ( 'NONE', #28739, 32.32717498572581860 ) ;
#15385=ORIENTED_EDGE ( 'NONE', *, *, #11161, .F. ) ;
#15396=DIRECTION ( 'NONE',  ( -0.000000000000000000, -0.000000000000000000, -1.000000000000000000 ) ) ;
#15409=FACE_OUTER_BOUND ( 'NONE', #4199, .T. ) ;
#15413=AXIS2_PLACEMENT_3D ( 'NONE', #9044, #23520, #4511 ) ;
#15414=DIRECTION ( 'NONE',  ( 1.000000000000000000, 0.000000000000000000, 0.000000000000000000 ) ) ;
#15421=VERTEX_POINT ( 'NONE', #9556 ) ;
#15442=CARTESIAN_POINT ( 'NONE',  ( 16.47768670952434178, 14.41708049311048789, 1.500000000000000000 ) ) ;
#15481=CYLINDRICAL_SURFACE ( 'NONE', #14980, 11.46182693247429718 ) ;
#15496=EDGE_CURVE ( 'NONE', #23725, #28435, #2710, .T. ) ;
#15512=ORIENTED_EDGE ( 'NONE', *, *, #7057, .T. ) ;
#15568=CYLINDRICAL_SURFACE ( 'NONE', #28311, 2.898871837527149165 ) ;
#15582=CARTESIAN_POINT ( 'NONE',  ( 0.000000000000000000, 0.000000000000000000, 1.500000000000000000 ) ) ;
#15589=VERTEX_POINT ( 'NONE', #613 ) ;
#15596=FACE_OUTER_BOUND ( 'NONE', #7978, .T. ) ;
#15603=CARTESIAN_POINT ( 'NONE',  ( -6.414842543015754295, -17.06554576617236307, 1.500000000000000000 ) ) ;
#15611=LINE ( 'NONE', #6256, #27273 ) ;
#15616=DIRECTION ( 'NONE',  ( 1.000000000000000000, 0.000000000000000000, 0.000000000000000000 ) ) ;
#15624=DIRECTION ( 'NONE',  ( -1.000000000000000000, 0.000000000000000000, 0.000000000000000000 ) ) ;
#15630=EDGE_CURVE ( 'NONE', #28141, #18363, #7967, .T. ) ;
#15636=DIRECTION ( 'NONE',  ( 0.000000000000000000, -0.000000000000000000, -1.000000000000000000 ) ) ;
#15657=CARTESIAN_POINT ( 'NONE',  ( -15.57266529552203416, 38.96488032230103471, -1.500000000000000000 ) ) ;
#15661=VECTOR ( 'NONE', #4042, 1000.000000000000000 ) ;
#15670=FACE_OUTER_BOUND ( 'NONE', #5889, .T. ) ;
#15681=DIRECTION ( 'NONE',  ( 0.4495526574063634095, -0.8932538319083086487, 0.000000000000000000 ) ) ;
#15705=CARTESIAN_POINT ( 'NONE',  ( -24.03057240117691862, -26.57182937991349903, -1.500000000000000000 ) ) ;
#15706=VECTOR ( 'NONE', #15120, 1000.000000000000000 ) ;
#15707=ORIENTED_EDGE ( 'NONE', *, *, #27710, .T. ) ;
#15715=CARTESIAN_POINT ( 'NONE',  ( 28.34828976096172681, -29.18752572968383419, 1.500000000000000000 ) ) ;
#15720=FACE_BOUND ( 'NONE', #15832, .T. ) ;
#15734=AXIS2_PLACEMENT_3D ( 'NONE', #25443, #20295, #22931 ) ;
#15762=EDGE_CURVE ( 'NONE', #6841, #2309, #25418, .T. ) ;
#15776=DIRECTION ( 'NONE',  ( -0.000000000000000000, 0.000000000000000000, 1.000000000000000000 ) ) ;
#15777=ORIENTED_EDGE ( 'NONE', *, *, #5581, .F. ) ;
#15778=CIRCLE ( 'NONE', #18765, 28.20443790117963800 ) ;
#15791=DIRECTION ( 'NONE',  ( -1.000000000000000000, 0.000000000000000000, 0.000000000000000000 ) ) ;
#15795=DIRECTION ( 'NONE',  ( -0.000000000000000000, -0.000000000000000000, -1.000000000000000000 ) ) ;
#15815=CARTESIAN_POINT ( 'NONE',  ( -4.163336342344337027E-14, 1.387778780781445676E-14, -1.500000000000000000 ) ) ;
#15820=CARTESIAN_POINT ( 'NONE',  ( -2.931009552726342449, 14.22630671667915792, 1.500000000000000000 ) ) ;
#15822=VERTEX_POINT ( 'NONE', #12140 ) ;
#15823=CIRCLE ( 'NONE', #19243, 1.447898107987198646 ) ;
#15832=EDGE_LOOP ( 'NONE', ( #17837, #6235, #13885, #8575, #27707 ) ) ;
#15836=DIRECTION ( 'NONE',  ( 1.000000000000000000, 0.000000000000000000, 0.000000000000000000 ) ) ;
#15837=CARTESIAN_POINT ( 'NONE',  ( -9.216505592218814158, -7.781333699927420966, 1.500000000000000000 ) ) ;
#15838=AXIS2_PLACEMENT_3D ( 'NONE', #15705, #13080, #12614 ) ;
#15839=EDGE_CURVE ( 'NONE', #24441, #24048, #11531, .T. ) ;
#15846=ADVANCED_FACE ( 'NONE', ( #6830 ), #26021, .T. ) ;
#15854=EDGE_CURVE ( 'NONE', #19170, #23449, #20648, .T. ) ;
#15856=EDGE_LOOP ( 'NONE', ( #10493, #15385, #22443, #14045 ) ) ;
#15857=VECTOR ( 'NONE', #30182, 1000.000000000000000 ) ;
#15871=CARTESIAN_POINT ( 'NONE',  ( 26.36764545593179676, 31.31467416275351923, 1.500000000000000000 ) ) ;
#15887=EDGE_CURVE ( 'NONE', #6434, #20068, #206, .T. ) ;
#15892=EDGE_LOOP ( 'NONE', ( #8175, #19242, #4618, #24074 ) ) ;
#15909=CARTESIAN_POINT ( 'NONE',  ( -15.10419704716067102, -17.26937953831884442, 1.500000000000000000 ) ) ;
#15914=EDGE_LOOP ( 'NONE', ( #25274, #24436, #5457, #19254 ) ) ;
#15919=ORIENTED_EDGE ( 'NONE', *, *, #20894, .T. ) ;
#15920=AXIS2_PLACEMENT_3D ( 'NONE', #24632, #3265, #10450 ) ;
#15924=DIRECTION ( 'NONE',  ( -0.000000000000000000, 0.000000000000000000, 1.000000000000000000 ) ) ;
#15926=CIRCLE ( 'NONE', #25383, 21.71568325578202163 ) ;
#15936=DIRECTION ( 'NONE',  ( -0.000000000000000000, -0.000000000000000000, -1.000000000000000000 ) ) ;
#15937=CARTESIAN_POINT ( 'NONE',  ( 17.26937953831880534, -14.36006998371588317, 1.500000000000000000 ) ) ;
#15941=CIRCLE ( 'NONE', #2480, 0.7441270634457163302 ) ;
#15961=DIRECTION ( 'NONE',  ( 1.000000000000000000, 0.000000000000000000, 0.000000000000000000 ) ) ;
#15998=CARTESIAN_POINT ( 'NONE',  ( -4.163336342344337027E-14, 1.387778780781445676E-14, 1.500000000000000000 ) ) ;
#16000=CARTESIAN_POINT ( 'NONE',  ( -4.163336342344337027E-14, -1.387778780781445676E-14, -1.500000000000000000 ) ) ;
#16015=VECTOR ( 'NONE', #30485, 1000.000000000000000 ) ;
#16025=ORIENTED_EDGE ( 'NONE', *, *, #6709, .T. ) ;
#16027=FACE_OUTER_BOUND ( 'NONE', #26194, .T. ) ;
#16057=ORIENTED_EDGE ( 'NONE', *, *, #18625, .F. ) ;
#16064=EDGE_CURVE ( 'NONE', #14826, #30777, #18190, .T. ) ;
#16088=DIRECTION ( 'NONE',  ( 1.000000000000000000, 0.000000000000000000, 0.000000000000000000 ) ) ;
#16092=DIRECTION ( 'NONE',  ( -0.000000000000000000, -0.000000000000000000, -1.000000000000000000 ) ) ;
#16108=CYLINDRICAL_SURFACE ( 'NONE', #6848, 37.60050224823048381 ) ;
#16113=ORIENTED_EDGE ( 'NONE', *, *, #4610, .T. ) ;
#16115=AXIS2_PLACEMENT_3D ( 'NONE', #15937, #29974, #30272 ) ;
#16118=VECTOR ( 'NONE', #11247, 1000.000000000000000 ) ;
#16122=EDGE_LOOP ( 'NONE', ( #29106, #25528, #9684, #17109 ) ) ;
#16166=CARTESIAN_POINT ( 'NONE',  ( 22.58267429318974706, -26.57182937991349903, 1.500000000000000000 ) ) ;
#16175=ORIENTED_EDGE ( 'NONE', *, *, #20617, .T. ) ;
#16178=DIRECTION ( 'NONE',  ( -1.000000000000000000, 0.000000000000000000, 0.000000000000000000 ) ) ;
#16179=CARTESIAN_POINT ( 'NONE',  ( 9.675133109038689838, -8.168544852422947145, 1.500000000000000000 ) ) ;
#16182=DIRECTION ( 'NONE',  ( -0.000000000000000000, -0.000000000000000000, -1.000000000000000000 ) ) ;
#16184=CARTESIAN_POINT ( 'NONE',  ( 15.57266529552203416, 38.96488032230103471, -1.500000000000000000 ) ) ;
#16193=ORIENTED_EDGE ( 'NONE', *, *, #9960, .T. ) ;
#16217=CARTESIAN_POINT ( 'NONE',  ( -3.221450758838616757, 1.621276839356792454, 1.500000000000000000 ) ) ;
#16221=EDGE_LOOP ( 'NONE', ( #16904, #18451, #14817, #10879 ) ) ;
#16223=DIRECTION ( 'NONE',  ( -0.000000000000000000, -0.000000000000000000, -1.000000000000000000 ) ) ;
#16226=CARTESIAN_POINT ( 'NONE',  ( -9.675133109038686285, -8.168544852422948921, 1.500000000000000000 ) ) ;
#16238=PLANE ( 'NONE',  #9829 ) ;
#16239=ORIENTED_EDGE ( 'NONE', *, *, #26518, .F. ) ;
#16253=EDGE_CURVE ( 'NONE', #8993, #25738, #17236, .T. ) ;
#16254=VERTEX_POINT ( 'NONE', #17082 ) ;
#16264=EDGE_CURVE ( 'NONE', #11996, #12516, #12189, .T. ) ;
#16280=VECTOR ( 'NONE', #7278, 1000.000000000000000 ) ;
#16297=DIRECTION ( 'NONE',  ( -0.000000000000000000, 0.000000000000000000, 1.000000000000000000 ) ) ;
#16303=DIRECTION ( 'NONE',  ( 0.000000000000000000, -0.000000000000000000, -1.000000000000000000 ) ) ;
#16312=AXIS2_PLACEMENT_3D ( 'NONE', #23633, #6807, #4313 ) ;
#16338=DIRECTION ( 'NONE',  ( -0.000000000000000000, -0.000000000000000000, -1.000000000000000000 ) ) ;
#16339=CARTESIAN_POINT ( 'NONE',  ( -2.931009552726342449, 14.22630671667915792, -1.500000000000000000 ) ) ;
#16359=VERTEX_POINT ( 'NONE', #7069 ) ;
#16366=ORIENTED_EDGE ( 'NONE', *, *, #6132, .T. ) ;
#16384=LINE ( 'NONE', #26051, #8649 ) ;
#16393=VERTEX_POINT ( 'NONE', #27984 ) ;
#16399=EDGE_LOOP ( 'NONE', ( #15088, #8291, #9992, #8075 ) ) ;
#16409=EDGE_CURVE ( 'NONE', #21650, #28935, #14180, .T. ) ;
#16420=DIRECTION ( 'NONE',  ( 1.000000000000000000, 0.000000000000000000, 0.000000000000000000 ) ) ;
#16442=EDGE_CURVE ( 'NONE', #8763, #16733, #1727, .T. ) ;
#16467=CARTESIAN_POINT ( 'NONE',  ( -13.88429941593315853, -16.69721919944146649, 1.500000000000000000 ) ) ;
#16481=AXIS2_PLACEMENT_3D ( 'NONE', #20506, #25181, #22678 ) ;
#16486=DIRECTION ( 'NONE',  ( -1.000000000000000000, 0.000000000000000000, 0.000000000000000000 ) ) ;
#16553=DIRECTION ( 'NONE',  ( 0.000000000000000000, -0.000000000000000000, -1.000000000000000000 ) ) ;
#16559=ADVANCED_FACE ( 'NONE', ( #26715 ), #26568, .F. ) ;
#16574=VECTOR ( 'NONE', #7567, 1000.000000000000000 ) ;
#16616=EDGE_CURVE ( 'NONE', #12630, #15107, #9228, .T. ) ;
#16630=EDGE_CURVE ( 'NONE', #9405, #29550, #20687, .T. ) ;
#16642=DIRECTION ( 'NONE',  ( -0.000000000000000000, -0.000000000000000000, -1.000000000000000000 ) ) ;
#16659=ORIENTED_EDGE ( 'NONE', *, *, #2117, .T. ) ;
#16669=AXIS2_PLACEMENT_3D ( 'NONE', #28670, #11987, #7150 ) ;
#16679=FACE_BOUND ( 'NONE', #18629, .T. ) ;
#16682=LINE ( 'NONE', #21337, #23195 ) ;
#16685=ORIENTED_EDGE ( 'NONE', *, *, #22321, .T. ) ;
#16698=DIRECTION ( 'NONE',  ( -1.000000000000000000, 0.000000000000000000, 0.000000000000000000 ) ) ;
#16709=DIRECTION ( 'NONE',  ( 1.000000000000000000, 0.000000000000000000, 0.000000000000000000 ) ) ;
#16711=ADVANCED_FACE ( 'NONE', ( #30283 ), #25905, .F. ) ;
#16718=CARTESIAN_POINT ( 'NONE',  ( 14.89473990422475680, -17.79239818699420539, 1.500000000000000000 ) ) ;
#16722=CARTESIAN_POINT ( 'NONE',  ( -17.22181377296915272, -14.41708049311147555, -1.500000000000000000 ) ) ;
#16730=ORIENTED_EDGE ( 'NONE', *, *, #652, .T. ) ;
#16733=VERTEX_POINT ( 'NONE', #28405 ) ;
#16754=PLANE ( 'NONE',  #14270 ) ;
#16765=CYLINDRICAL_SURFACE ( 'NONE', #2940, 0.6002263538043648428 ) ;
#16767=VERTEX_POINT ( 'NONE', #11565 ) ;
#16779=ORIENTED_EDGE ( 'NONE', *, *, #5011, .F. ) ;
#16785=VECTOR ( 'NONE', #24033, 1000.000000000000000 ) ;
#16797=CARTESIAN_POINT ( 'NONE',  ( 28.34828976096172681, 29.18752572968383419, -1.500000000000000000 ) ) ;
#16799=VERTEX_POINT ( 'NONE', #14970 ) ;
#16806=EDGE_CURVE ( 'NONE', #584, #30261, #5250, .T. ) ;
#16812=CIRCLE ( 'NONE', #4875, 23.20393738267408779 ) ;
#16813=DIRECTION ( 'NONE',  ( 1.000000000000000000, 0.000000000000000000, 0.000000000000000000 ) ) ;
#16815=AXIS2_PLACEMENT_3D ( 'NONE', #6405, #15924, #1108 ) ;
#16837=FACE_BOUND ( 'NONE', #3542, .T. ) ;
#16846=DIRECTION ( 'NONE',  ( -0.000000000000000000, -0.000000000000000000, -1.000000000000000000 ) ) ;
#16875=CARTESIAN_POINT ( 'NONE',  ( 26.36764545593179676, 31.31467416275351923, 1.500000000000000000 ) ) ;
#16876=CIRCLE ( 'NONE', #19303, 32.32717498572574755 ) ;
#16891=EDGE_CURVE ( 'NONE', #25685, #24048, #23336, .T. ) ;
#16894=AXIS2_PLACEMENT_3D ( 'NONE', #23430, #28289, #1632 ) ;
#16904=ORIENTED_EDGE ( 'NONE', *, *, #8197, .T. ) ;
#16911=CARTESIAN_POINT ( 'NONE',  ( -8.757878075398936701, -7.394122547431892123, -1.500000000000000000 ) ) ;
#16953=ORIENTED_EDGE ( 'NONE', *, *, #13604, .F. ) ;
#16956=ORIENTED_EDGE ( 'NONE', *, *, #28037, .F. ) ;
#16967=CARTESIAN_POINT ( 'NONE',  ( 1.073881485057758711, 0.9711784013061475207, 1.500000000000000000 ) ) ;
#16972=EDGE_CURVE ( 'NONE', #27445, #25738, #19688, .T. ) ;
#16984=CIRCLE ( 'NONE', #29451, 2.898871837527151385 ) ;
#17025=CARTESIAN_POINT ( 'NONE',  ( 11.21147646446735102, -30.29926891764210595, 1.500000000000000000 ) ) ;
#17027=DIRECTION ( 'NONE',  ( -0.000000000000000000, 0.000000000000000000, 1.000000000000000000 ) ) ;
#17036=CYLINDRICAL_SURFACE ( 'NONE', #8002, 32.32717498572574755 ) ;
#17041=ORIENTED_EDGE ( 'NONE', *, *, #7124, .T. ) ;
#17058=FACE_OUTER_BOUND ( 'NONE', #14692, .T. ) ;
#17074=ORIENTED_EDGE ( 'NONE', *, *, #24890, .T. ) ;
#17082=CARTESIAN_POINT ( 'NONE',  ( -22.95669091611927826, -27.54300778121952220, -1.500000000000000000 ) ) ;
#17096=CYLINDRICAL_SURFACE ( 'NONE', #423, 23.20393738267338790 ) ;
#17109=ORIENTED_EDGE ( 'NONE', *, *, #63, .F. ) ;
#17120=PLANE ( 'NONE',  #12291 ) ;
#17126=CIRCLE ( 'NONE', #6666, 1.447898107987170890 ) ;
#17131=CARTESIAN_POINT ( 'NONE',  ( -23.17581250239728519, 34.50630206824671831, -1.499999999999999778 ) ) ;
#17136=ORIENTED_EDGE ( 'NONE', *, *, #17400, .F. ) ;
#17168=CARTESIAN_POINT ( 'NONE',  ( -2.931009552726339784, -14.22630671667915969, 1.500000000000000000 ) ) ;
#17186=EDGE_CURVE ( 'NONE', #19170, #27254, #23729, .T. ) ;
#17192=ORIENTED_EDGE ( 'NONE', *, *, #20131, .T. ) ;
#17231=DIRECTION ( 'NONE',  ( -0.000000000000000000, -0.000000000000000000, -1.000000000000000000 ) ) ;
#17236=LINE ( 'NONE', #5392, #26143 ) ;
#17241=EDGE_CURVE ( 'NONE', #20990, #10442, #13254, .T. ) ;
#17246=CARTESIAN_POINT ( 'NONE',  ( 0.000000000000000000, 0.000000000000000000, 1.500000000000000000 ) ) ;
#17249=AXIS2_PLACEMENT_3D ( 'NONE', #2079, #18941, #2234 ) ;
#17263=DIRECTION ( 'NONE',  ( -0.000000000000000000, -0.000000000000000000, -1.000000000000000000 ) ) ;
#17264=ORIENTED_EDGE ( 'NONE', *, *, #5011, .T. ) ;
#17278=DIRECTION ( 'NONE',  ( -0.000000000000000000, -0.000000000000000000, -1.000000000000000000 ) ) ;
#17282=ORIENTED_EDGE ( 'NONE', *, *, #22693, .T. ) ;
#17297=CIRCLE ( 'NONE', #1871, 37.60050224823048381 ) ;
#17309=CIRCLE ( 'NONE', #16312, 28.20443790117971261 ) ;
#17310=LINE ( 'NONE', #19965, #17406 ) ;
#17322=PLANE ( 'NONE',  #17858 ) ;
#17332=CARTESIAN_POINT ( 'NONE',  ( -16.65122935894506639, -13.93942108199812324, 1.500000000000000000 ) ) ;
#17335=VERTEX_POINT ( 'NONE', #12199 ) ;
#17344=LINE ( 'NONE', #10166, #19810 ) ;
#17351=DIRECTION ( 'NONE',  ( 1.000000000000000000, 1.776356839400250465E-15, 0.000000000000000000 ) ) ;
#17352=ORIENTED_EDGE ( 'NONE', *, *, #21768, .T. ) ;
#17370=EDGE_CURVE ( 'NONE', #22982, #6819, #5781, .T. ) ;
#17396=SHAPE_DEFINITION_REPRESENTATION ( #28862, #7129 ) ;
#17400=EDGE_CURVE ( 'NONE', #8016, #27429, #26703, .T. ) ;
#17406=VECTOR ( 'NONE', #29483, 1000.000000000000000 ) ;
#17413=DIRECTION ( 'NONE',  ( -1.000000000000000000, 0.000000000000000000, 0.000000000000000000 ) ) ;
#17415=CARTESIAN_POINT ( 'NONE',  ( -4.163336342344337027E-14, 1.387778780781445676E-14, 1.500000000000000000 ) ) ;
#17416=ORIENTED_EDGE ( 'NONE', *, *, #5172, .T. ) ;
#17420=CARTESIAN_POINT ( 'NONE',  ( -4.163336342344337027E-14, 1.387778780781445676E-14, 1.500000000000000000 ) ) ;
#17421=CARTESIAN_POINT ( 'NONE',  ( 28.37932450449293853, 10.51822134874671022, -1.500000000000000000 ) ) ;
#17428=AXIS2_PLACEMENT_3D ( 'NONE', #21092, #4125, #6922 ) ;
#17435=EDGE_CURVE ( 'NONE', #3576, #3847, #8259, .T. ) ;
#17437=AXIS2_PLACEMENT_3D ( 'NONE', #4294, #7104, #11629 ) ;
#17457=CARTESIAN_POINT ( 'NONE',  ( 17.26937953831880534, -14.36006998371588317, -1.500000000000000000 ) ) ;
#17463=DIRECTION ( 'NONE',  ( -0.4495526574063634095, -0.8932538319083086487, 0.000000000000000000 ) ) ;
#17468=CARTESIAN_POINT ( 'NONE',  ( 43.34097750826428097, 11.89502811014149763, -1.500000000000000444 ) ) ;
#17473=CARTESIAN_POINT ( 'NONE',  ( -15.16120755655624741, 17.22181377296911720, 1.500000000000000000 ) ) ;
#17495=ORIENTED_EDGE ( 'NONE', *, *, #15496, .F. ) ;
#17500=ORIENTED_EDGE ( 'NONE', *, *, #11301, .F. ) ;
#17510=VECTOR ( 'NONE', #27862, 1000.000000000000000 ) ;
#17534=EDGE_CURVE ( 'NONE', #27429, #584, #14744, .T. ) ;
#17540=ORIENTED_EDGE ( 'NONE', *, *, #27469, .T. ) ;
#17541=CARTESIAN_POINT ( 'NONE',  ( -3.221450758838616757, -1.621276839356792454, 1.500000000000000000 ) ) ;
#17555=ORIENTED_EDGE ( 'NONE', *, *, #24844, .F. ) ;
#17556=CARTESIAN_POINT ( 'NONE',  ( 8.860628911697515875, 8.184276679720483116, 1.500000000000000000 ) ) ;
#17575=CARTESIAN_POINT ( 'NONE',  ( -4.163336342344337027E-14, 1.387778780781445676E-14, -1.500000000000000000 ) ) ;
#17577=ORIENTED_EDGE ( 'NONE', *, *, #23411, .F. ) ;
#17578=CARTESIAN_POINT ( 'NONE',  ( -13.88429941593315853, -16.69721919944146649, -1.500000000000000000 ) ) ;
#17583=EDGE_CURVE ( 'NONE', #18859, #21029, #26041, .T. ) ;
#17585=EDGE_CURVE ( 'NONE', #17335, #16359, #16682, .T. ) ;
#17589=CIRCLE ( 'NONE', #4137, 0.7441270634457319844 ) ;
#17596=ORIENTED_EDGE ( 'NONE', *, *, #17370, .T. ) ;
#17639=ORIENTED_EDGE ( 'NONE', *, *, #22496, .T. ) ;
#17641=DIRECTION ( 'NONE',  ( 1.000000000000000000, 0.000000000000000000, 0.000000000000000000 ) ) ;
#17675=CARTESIAN_POINT ( 'NONE',  ( 28.37932450449293853, 10.51822134874671022, 1.500000000000000000 ) ) ;
#17681=ORIENTED_EDGE ( 'NONE', *, *, #30016, .F. ) ;
#17685=DIRECTION ( 'NONE',  ( -1.000000000000000000, 0.000000000000000000, 0.000000000000000000 ) ) ;
#17690=( BOUNDED_SURFACE ( )  B_SPLINE_SURFACE ( 3, 1, ( 
 ( #20111, #7640 ),
 ( #12487, #5760 ),
 ( #10279, #17468 ),
 ( #12325, #5296 ) ),
 .UNSPECIFIED., .F., .F., .T. ) 
 B_SPLINE_SURFACE_WITH_KNOTS ( ( 4, 4 ),
 ( 2, 2 ),
 ( 0.000000000000000000, 1.000000000000000000 ),
 ( 0.000000000000000000, 1.000000000000000000 ),
 .UNSPECIFIED. ) 
 GEOMETRIC_REPRESENTATION_ITEM ( )  RATIONAL_B_SPLINE_SURFACE ( (
 ( 1.000000000000000000, 1.000000000000000000),
 ( 0.8179194830933627092, 0.8179194830933627092),
 ( 0.8179194830933627092, 0.8179194830933627092),
 ( 1.000000000000000000, 1.000000000000000000) ) ) 
 REPRESENTATION_ITEM ( '' )  SURFACE ( )  );
#17692=AXIS2_PLACEMENT_3D ( 'NONE', #3947, #22950, #11113 ) ;
#17698=EDGE_LOOP ( 'NONE', ( #28882, #19147, #24057, #18065 ) ) ;
#17699=DIRECTION ( 'NONE',  ( 0.6707505147970024284, 0.7416830501633134842, 0.000000000000000000 ) ) ;
#17702=ORIENTED_EDGE ( 'NONE', *, *, #22687, .T. ) ;
#17718=LINE ( 'NONE', #12283, #1135 ) ;
#17722=CARTESIAN_POINT ( 'NONE',  ( -8.419710366748644148, 7.777014463793872956, 1.500000000000000000 ) ) ;
#17755=CIRCLE ( 'NONE', #12286, 10.00000000000000000 ) ;
#17763=AXIS2_PLACEMENT_3D ( 'NONE', #666, #7850, #21565 ) ;
#17765=ORIENTED_EDGE ( 'NONE', *, *, #26117, .F. ) ;
#17766=ORIENTED_EDGE ( 'NONE', *, *, #10561, .T. ) ;
#17781=EDGE_CURVE ( 'NONE', #8016, #14669, #19733, .T. ) ;
#17785=EDGE_CURVE ( 'NONE', #6787, #2517, #1821, .T. ) ;
#17823=CYLINDRICAL_SURFACE ( 'NONE', #25342, 10.00000000000000000 ) ;
#17837=ORIENTED_EDGE ( 'NONE', *, *, #2110, .F. ) ;
#17841=FACE_OUTER_BOUND ( 'NONE', #22524, .T. ) ;
#17845=CARTESIAN_POINT ( 'NONE',  ( 15.57266529552203416, -38.96488032230103471, 1.500000000000000000 ) ) ;
#17849=ORIENTED_EDGE ( 'NONE', *, *, #25426, .F. ) ;
#17850=VECTOR ( 'NONE', #2528, 1000.000000000000000 ) ;
#17858=AXIS2_PLACEMENT_3D ( 'NONE', #26852, #5778, #12808 ) ;
#17865=ORIENTED_EDGE ( 'NONE', *, *, #1172, .T. ) ;
#17888=( BOUNDED_CURVE ( )  B_SPLINE_CURVE ( 3, ( #2567, #18791, #213, #9726 ),
 .UNSPECIFIED., .F., .T. ) 
 B_SPLINE_CURVE_WITH_KNOTS ( ( 4, 4 ),
 ( 2.399144907686414196, 2.730840413552699353 ),
 .UNSPECIFIED. ) 
 CURVE ( )  GEOMETRIC_REPRESENTATION_ITEM ( )  RATIONAL_B_SPLINE_CURVE ( ( 1.000000000000000000, 0.9908525036704132205, 0.9908525036704132205, 1.000000000000000000 ) ) 
 REPRESENTATION_ITEM ( '' )  );
#17893=PRODUCT_DEFINITION_FORMATION_WITH_SPECIFIED_SOURCE ( 'ANY', '', #14916, .NOT_KNOWN. ) ;
#17905=ORIENTED_EDGE ( 'NONE', *, *, #20232, .F. ) ;
#17928=ORIENTED_EDGE ( 'NONE', *, *, #22726, .T. ) ;
#17935=EDGE_LOOP ( 'NONE', ( #26077, #21056, #1743, #7789, #9236, #23814 ) ) ;
#17958=ORIENTED_EDGE ( 'NONE', *, *, #19493, .T. ) ;
#17962=ADVANCED_FACE ( 'NONE', ( #12745 ), #24281, .F. ) ;
#17977=DIRECTION ( 'NONE',  ( -0.000000000000000000, -0.000000000000000000, -1.000000000000000000 ) ) ;
#17978=CARTESIAN_POINT ( 'NONE',  ( 25.10445388623454477, 25.60065097860747585, 1.500000000000000000 ) ) ;
#17985=DIRECTION ( 'NONE',  ( -0.000000000000000000, 0.000000000000000000, 1.000000000000000000 ) ) ;
#18016=CARTESIAN_POINT ( 'NONE',  ( -4.163336342344337027E-14, -1.387778780781445676E-14, -1.500000000000000000 ) ) ;
#18023=ORIENTED_EDGE ( 'NONE', *, *, #8754, .T. ) ;
#18029=EDGE_CURVE ( 'NONE', #4388, #8400, #8071, .T. ) ;
#18033=CARTESIAN_POINT ( 'NONE',  ( 15.57266529552203416, 38.96488032230103471, 1.500000000000000000 ) ) ;
#18036=DIRECTION ( 'NONE',  ( -0.000000000000000000, 0.000000000000000000, 1.000000000000000000 ) ) ;
#18065=ORIENTED_EDGE ( 'NONE', *, *, #10385, .T. ) ;
#18080=DIRECTION ( 'NONE',  ( 0.000000000000000000, -0.000000000000000000, -1.000000000000000000 ) ) ;
#18105=ORIENTED_EDGE ( 'NONE', *, *, #26149, .T. ) ;
#18129=ORIENTED_EDGE ( 'NONE', *, *, #16972, .F. ) ;
#18131=CYLINDRICAL_SURFACE ( 'NONE', #12674, 0.7441270634457337607 ) ;
#18148=CARTESIAN_POINT ( 'NONE',  ( 22.95669091611928181, 27.54300778121952575, 1.500000000000000000 ) ) ;
#18160=CARTESIAN_POINT ( 'NONE',  ( 0.000000000000000000, -5.590849009245238754, -1.500000000000000000 ) ) ;
#18161=ORIENTED_EDGE ( 'NONE', *, *, #251, .T. ) ;
#18189=DIRECTION ( 'NONE',  ( 1.000000000000000000, 0.000000000000000000, 0.000000000000000000 ) ) ;
#18190=CIRCLE ( 'NONE', #10699, 1.447898107987198646 ) ;
#18200=LINE ( 'NONE', #4465, #26853 ) ;
#18211=ORIENTED_EDGE ( 'NONE', *, *, #21582, .T. ) ;
#18219=CARTESIAN_POINT ( 'NONE',  ( 17.26937953831880534, -14.36006998371588317, 1.500000000000000000 ) ) ;
#18227=ORIENTED_EDGE ( 'NONE', *, *, #19668, .T. ) ;
#18247=ORIENTED_EDGE ( 'NONE', *, *, #20232, .T. ) ;
#18248=DIRECTION ( 'NONE',  ( -0.000000000000000000, 0.000000000000000000, 1.000000000000000000 ) ) ;
#18282=CIRCLE ( 'NONE', #12807, 21.71568325578193637 ) ;
#18286=ORIENTED_EDGE ( 'NONE', *, *, #9245, .F. ) ;
#18298=DIRECTION ( 'NONE',  ( -0.000000000000000000, 0.000000000000000000, 1.000000000000000000 ) ) ;
#18330=ORIENTED_EDGE ( 'NONE', *, *, #3242, .F. ) ;
#18333=DIRECTION ( 'NONE',  ( -0.000000000000000000, 0.000000000000000000, 1.000000000000000000 ) ) ;
#18339=AXIS2_PLACEMENT_3D ( 'NONE', #1914, #23569, #1625 ) ;
#18340=CARTESIAN_POINT ( 'NONE',  ( -14.83584055149731817, -17.84153987719691514, 1.500000000000000000 ) ) ;
#18360=VECTOR ( 'NONE', #5761, 1000.000000000000000 ) ;
#18361=LINE ( 'NONE', #16467, #28340 ) ;
#18363=VERTEX_POINT ( 'NONE', #9083 ) ;
#18373=AXIS2_PLACEMENT_3D ( 'NONE', #1138, #27353, #5510 ) ;
#18388=LINE ( 'NONE', #15020, #29542 ) ;
#18405=LINE ( 'NONE', #6223, #24565 ) ;
#18424=CARTESIAN_POINT ( 'NONE',  ( -2.931009552726342449, 14.22630671667915792, 1.500000000000000000 ) ) ;
#18428=AXIS2_PLACEMENT_3D ( 'NONE', #24992, #10805, #3317 ) ;
#18432=ORIENTED_EDGE ( 'NONE', *, *, #12611, .F. ) ;
#18451=ORIENTED_EDGE ( 'NONE', *, *, #19285, .T. ) ;
#18456=ORIENTED_EDGE ( 'NONE', *, *, #25356, .T. ) ;
#18463=DIRECTION ( 'NONE',  ( -0.000000000000000000, -0.000000000000000000, -1.000000000000000000 ) ) ;
#18469=CARTESIAN_POINT ( 'NONE',  ( -11.21147646446735102, -30.29926891764210595, 1.500000000000000000 ) ) ;
#18477=DIRECTION ( 'NONE',  ( 0.000000000000000000, -0.000000000000000000, -1.000000000000000000 ) ) ;
#18478=ORIENTED_EDGE ( 'NONE', *, *, #15839, .F. ) ;
#18483=ORIENTED_EDGE ( 'NONE', *, *, #24018, .F. ) ;
#18488=DIRECTION ( 'NONE',  ( -0.000000000000000000, -0.000000000000000000, -1.000000000000000000 ) ) ;
#18496=AXIS2_PLACEMENT_3D ( 'NONE', #4240, #6278, #25149 ) ;
#18501=DIRECTION ( 'NONE',  ( 1.000000000000000000, 0.000000000000000000, 0.000000000000000000 ) ) ;
#18511=LINE ( 'NONE', #7107, #27345 ) ;
#18522=DIRECTION ( 'NONE',  ( -0.6707505147970023174, 0.7416830501633134842, 0.000000000000000000 ) ) ;
#18524=ADVANCED_FACE ( 'NONE', ( #21683 ), #322, .F. ) ;
#18529=EDGE_CURVE ( 'NONE', #19397, #12669, #17755, .T. ) ;
#18552=CARTESIAN_POINT ( 'NONE',  ( -19.54426622602688113, 37.07991288358297055, -1.499999999999999778 ) ) ;
#18556=ADVANCED_FACE ( 'NONE', ( #15596 ), #1427, .F. ) ;
#18559=ADVANCED_FACE ( 'NONE', ( #29648 ), #26305, .F. ) ;
#18561=EDGE_CURVE ( 'NONE', #10191, #21504, #9307, .T. ) ;
#18612=DIRECTION ( 'NONE',  ( -0.000000000000000000, 0.000000000000000000, 1.000000000000000000 ) ) ;
#18625=EDGE_CURVE ( 'NONE', #21717, #9927, #29425, .T. ) ;
#18629=EDGE_LOOP ( 'NONE', ( #1304, #22032, #4630, #24711, #16366 ) ) ;
#18633=LINE ( 'NONE', #1788, #3923 ) ;
#18636=DIRECTION ( 'NONE',  ( -0.000000000000000000, 0.000000000000000000, 1.000000000000000000 ) ) ;
#18640=CARTESIAN_POINT ( 'NONE',  ( 26.83043119477639138, -8.695877139419035728, 1.500000000000000000 ) ) ;
#18644=CYLINDRICAL_SURFACE ( 'NONE', #6799, 0.6002263538043630664 ) ;
#18670=ORIENTED_EDGE ( 'NONE', *, *, #17534, .F. ) ;
#18674=CARTESIAN_POINT ( 'NONE',  ( 11.21147646446735102, -30.29926891764210595, -1.500000000000000000 ) ) ;
#18689=( BOUNDED_SURFACE ( )  B_SPLINE_SURFACE ( 3, 1, ( 
 ( #4976, #19166 ),
 ( #2791, #22116 ),
 ( #14951, #17131 ),
 ( #10262, #28686 ) ),
 .UNSPECIFIED., .F., .F., .T. ) 
 B_SPLINE_SURFACE_WITH_KNOTS ( ( 4, 4 ),
 ( 2, 2 ),
 ( 0.000000000000000000, 1.000000000000000000 ),
 ( 0.000000000000000000, 1.000000000000000000 ),
 .UNSPECIFIED. ) 
 GEOMETRIC_REPRESENTATION_ITEM ( )  RATIONAL_B_SPLINE_SURFACE ( (
 ( 1.000000000000000000, 1.000000000000000000),
 ( 0.9908525036704132205, 0.9908525036704132205),
 ( 0.9908525036704132205, 0.9908525036704132205),
 ( 1.000000000000000000, 1.000000000000000000) ) ) 
 REPRESENTATION_ITEM ( '' )  SURFACE ( )  );
#18694=ADVANCED_FACE ( 'NONE', ( #5408 ), #15054, .T. ) ;
#18696=CARTESIAN_POINT ( 'NONE',  ( 3.637110358602580362, -19.99473753024311762, -1.500000000000000000 ) ) ;
#18700=DIRECTION ( 'NONE',  ( 1.000000000000000000, 4.440892098500626162E-15, 0.000000000000000000 ) ) ;
#18706=DIRECTION ( 'NONE',  ( -0.6707505147970024284, -0.7416830501633134842, 0.000000000000000000 ) ) ;
#18729=DIRECTION ( 'NONE',  ( 1.000000000000000000, 0.000000000000000000, 0.000000000000000000 ) ) ;
#18737=DIRECTION ( 'NONE',  ( -0.8932538319083086487, 0.4495526574063634095, 0.000000000000000000 ) ) ;
#18749=STYLED_ITEM('',(#30886),#2768);
#18755=DIRECTION ( 'NONE',  ( 1.000000000000000000, 0.000000000000000000, 0.000000000000000000 ) ) ;
#18759=ORIENTED_EDGE ( 'NONE', *, *, #18561, .F. ) ;
#18765=AXIS2_PLACEMENT_3D ( 'NONE', #10696, #6019, #29725 ) ;
#18782=AXIS2_PLACEMENT_3D ( 'NONE', #26219, #19365, #19199 ) ;
#18787=AXIS2_PLACEMENT_3D ( 'NONE', #5295, #14803, #2970 ) ;
#18791=CARTESIAN_POINT ( 'NONE',  ( -23.17581250239728519, -34.50630206824673252, -1.499999999999999778 ) ) ;
#18820=DIRECTION ( 'NONE',  ( -0.000000000000000000, -0.000000000000000000, -1.000000000000000000 ) ) ;
#18839=CYLINDRICAL_SURFACE ( 'NONE', #25714, 0.7441270634457181066 ) ;
#18856=ORIENTED_EDGE ( 'NONE', *, *, #23411, .T. ) ;
#18859=VERTEX_POINT ( 'NONE', #18033 ) ;
#18877=DIRECTION ( 'NONE',  ( -0.4495526574063634095, -0.8932538319083086487, 0.000000000000000000 ) ) ;
#18881=( BOUNDED_SURFACE ( )  B_SPLINE_SURFACE ( 3, 1, ( 
 ( #13958, #2412 ),
 ( #23453, #28316 ),
 ( #21108, #25965 ),
 ( #4592, #23602 ) ),
 .UNSPECIFIED., .F., .F., .T. ) 
 B_SPLINE_SURFACE_WITH_KNOTS ( ( 4, 4 ),
 ( 2, 2 ),
 ( 0.000000000000000000, 1.000000000000000000 ),
 ( 0.000000000000000000, 1.000000000000000000 ),
 .UNSPECIFIED. ) 
 GEOMETRIC_REPRESENTATION_ITEM ( )  RATIONAL_B_SPLINE_SURFACE ( (
 ( 1.000000000000000000, 1.000000000000000000),
 ( 0.9908525036704132205, 0.9908525036704132205),
 ( 0.9908525036704132205, 0.9908525036704132205),
 ( 1.000000000000000000, 1.000000000000000000) ) ) 
 REPRESENTATION_ITEM ( '' )  SURFACE ( )  );
#18893=VERTEX_POINT ( 'NONE', #16911 ) ;
#18919=DIRECTION ( 'NONE',  ( 1.000000000000000000, -5.780230957810361426E-15, 0.000000000000000000 ) ) ;
#18941=DIRECTION ( 'NONE',  ( -0.000000000000000000, 0.000000000000000000, 1.000000000000000000 ) ) ;
#18963=EDGE_CURVE ( 'NONE', #4466, #8993, #17888, .T. ) ;
#18964=CARTESIAN_POINT ( 'NONE',  ( -23.20393738267338790, 0.000000000000000000, -1.500000000000000000 ) ) ;
#18970=DIRECTION ( 'NONE',  ( -0.000000000000000000, -0.000000000000000000, -1.000000000000000000 ) ) ;
#18983=VECTOR ( 'NONE', #28417, 1000.000000000000000 ) ;
#18985=AXIS2_PLACEMENT_3D ( 'NONE', #3983, #18333, #27847 ) ;
#18989=DIRECTION ( 'NONE',  ( 1.000000000000000000, 0.000000000000000000, 0.000000000000000000 ) ) ;
#18992=DIRECTION ( 'NONE',  ( -1.000000000000000000, 0.000000000000000000, 0.000000000000000000 ) ) ;
#19035=DIRECTION ( 'NONE',  ( -0.000000000000000000, -0.000000000000000000, -1.000000000000000000 ) ) ;
#19062=CARTESIAN_POINT ( 'NONE',  ( -3.515970705488605130, -17.06554576617236307, -1.500000000000000000 ) ) ;
#19064=CARTESIAN_POINT ( 'NONE',  ( -2.931009552726339784, -14.22630671667915969, -1.500000000000000000 ) ) ;
#19070=CARTESIAN_POINT ( 'NONE',  ( 0.000000000000000000, 0.000000000000000000, -1.500000000000000000 ) ) ;
#19077=CARTESIAN_POINT ( 'NONE',  ( -28.34828976096172326, 29.18752572968383063, 1.500000000000000000 ) ) ;
#19078=VERTEX_POINT ( 'NONE', #25146 ) ;
#19084=ORIENTED_EDGE ( 'NONE', *, *, #3095, .T. ) ;
#19091=ORIENTED_EDGE ( 'NONE', *, *, #25952, .T. ) ;
#19127=CARTESIAN_POINT ( 'NONE',  ( -28.37932450449293853, 10.51822134874671022, 1.500000000000000000 ) ) ;
#19137=CARTESIAN_POINT ( 'NONE',  ( 16.65122935894595813, 13.93942108199718888, 1.500000000000000000 ) ) ;
#19147=ORIENTED_EDGE ( 'NONE', *, *, #23433, .F. ) ;
#19159=ORIENTED_EDGE ( 'NONE', *, *, #14766, .F. ) ;
#19166=CARTESIAN_POINT ( 'NONE',  ( -15.57266529552203416, 38.96488032230103471, -1.500000000000000000 ) ) ;
#19170=VERTEX_POINT ( 'NONE', #22722 ) ;
#19187=DIRECTION ( 'NONE',  ( -0.000000000000000000, -0.000000000000000000, -1.000000000000000000 ) ) ;
#19199=DIRECTION ( 'NONE',  ( 1.000000000000000000, -2.396195514597832977E-15, 0.000000000000000000 ) ) ;
#19201=DIRECTION ( 'NONE',  ( 1.000000000000000000, 0.000000000000000000, 0.000000000000000000 ) ) ;
#19242=ORIENTED_EDGE ( 'NONE', *, *, #3095, .F. ) ;
#19243=AXIS2_PLACEMENT_3D ( 'NONE', #22074, #20048, #708 ) ;
#19248=DIRECTION ( 'NONE',  ( -0.4495526574063634095, 0.8932538319083086487, 0.000000000000000000 ) ) ;
#19249=DIRECTION ( 'NONE',  ( -0.000000000000000000, 0.000000000000000000, 1.000000000000000000 ) ) ;
#19250=EDGE_CURVE ( 'NONE', #9427, #22347, #733, .T. ) ;
#19254=ORIENTED_EDGE ( 'NONE', *, *, #26046, .F. ) ;
#19260=CYLINDRICAL_SURFACE ( 'NONE', #28518, 0.7441270634457337607 ) ;
#19270=CARTESIAN_POINT ( 'NONE',  ( -26.44644203219470668, 9.801837641955994940, 1.500000000000000000 ) ) ;
#19280=EDGE_LOOP ( 'NONE', ( #2980, #4825, #30560, #25652 ) ) ;
#19285=EDGE_CURVE ( 'NONE', #19397, #1725, #9303, .T. ) ;
#19297=AXIS2_PLACEMENT_3D ( 'NONE', #22440, #22127, #26834 ) ;
#19303=AXIS2_PLACEMENT_3D ( 'NONE', #5371, #23927, #28469 ) ;
#19307=CARTESIAN_POINT ( 'NONE',  ( -3.515970705488605130, 17.06554576617236307, 1.500000000000000000 ) ) ;
#19315=CARTESIAN_POINT ( 'NONE',  ( -15.57266529552203416, 38.96488032230103471, 1.500000000000000000 ) ) ;
#19323=VECTOR ( 'NONE', #24346, 1000.000000000000000 ) ;
#19324=EDGE_CURVE ( 'NONE', #6974, #22885, #17309, .T. ) ;
#19336=ORIENTED_EDGE ( 'NONE', *, *, #11860, .T. ) ;
#19357=EDGE_CURVE ( 'NONE', #3847, #5226, #4022, .T. ) ;
#19365=DIRECTION ( 'NONE',  ( 0.000000000000000000, -0.000000000000000000, -1.000000000000000000 ) ) ;
#19370=CARTESIAN_POINT ( 'NONE',  ( 26.36764545593179676, 31.31467416275351923, -1.500000000000000000 ) ) ;
#19390=CARTESIAN_POINT ( 'NONE',  ( -28.34828976096172326, 29.18752572968383063, -1.500000000000000000 ) ) ;
#19394=VERTEX_POINT ( 'NONE', #1831 ) ;
#19397=VERTEX_POINT ( 'NONE', #11356 ) ;
#19414=CARTESIAN_POINT ( 'NONE',  ( -14.41708049311053053, 17.22181377296911720, 1.500000000000000000 ) ) ;
#19420=CARTESIAN_POINT ( 'NONE',  ( 9.675133109038689838, -8.168544852422947145, -1.500000000000000000 ) ) ;
#19427=VERTEX_POINT ( 'NONE', #9012 ) ;
#19444=DIRECTION ( 'NONE',  ( -0.000000000000000000, 0.000000000000000000, 1.000000000000000000 ) ) ;
#19447=FACE_OUTER_BOUND ( 'NONE', #20176, .T. ) ;
#19472=ADVANCED_FACE ( 'NONE', ( #30823 ), #24107, .F. ) ;
#19493=EDGE_CURVE ( 'NONE', #26671, #20990, #22534, .T. ) ;
#19517=DIRECTION ( 'NONE',  ( -0.000000000000000000, -0.000000000000000000, -1.000000000000000000 ) ) ;
#19518=CARTESIAN_POINT ( 'NONE',  ( -23.17581250239728519, -34.50630206824672541, 1.499999999999999778 ) ) ;
#19520=ORIENTED_EDGE ( 'NONE', *, *, #22532, .T. ) ;
#19553=ORIENTED_EDGE ( 'NONE', *, *, #28807, .F. ) ;
#19556=CARTESIAN_POINT ( 'NONE',  ( 2.599508007902112006, -14.29059753516471964, 1.500000000000000000 ) ) ;
#19558=EDGE_LOOP ( 'NONE', ( #29861, #10013, #9424, #26717 ) ) ;
#19563=AXIS2_PLACEMENT_3D ( 'NONE', #12508, #7665, #17641 ) ;
#19567=DIRECTION ( 'NONE',  ( -0.000000000000000000, -0.000000000000000000, -1.000000000000000000 ) ) ;
#19574=ORIENTED_EDGE ( 'NONE', *, *, #11161, .T. ) ;
#19581=CARTESIAN_POINT ( 'NONE',  ( 15.57266529552203416, -38.96488032230103471, -1.500000000000000000 ) ) ;
#19588=DIRECTION ( 'NONE',  ( -1.000000000000000000, 0.000000000000000000, 0.000000000000000000 ) ) ;
#19605=CARTESIAN_POINT ( 'NONE',  ( 24.03057240117691862, -26.57182937991349903, 1.500000000000000000 ) ) ;
#19608=ORIENTED_EDGE ( 'NONE', *, *, #20284, .T. ) ;
#19617=ORIENTED_EDGE ( 'NONE', *, *, #4610, .F. ) ;
#19630=EDGE_LOOP ( 'NONE', ( #10247, #30082, #14736, #9717, #26739, #442 ) ) ;
#19640=VERTEX_POINT ( 'NONE', #19908 ) ;
#19655=DIRECTION ( 'NONE',  ( 1.000000000000000000, 0.000000000000000000, 0.000000000000000000 ) ) ;
#19656=DIRECTION ( 'NONE',  ( -1.000000000000000000, 0.000000000000000000, 0.000000000000000000 ) ) ;
#19668=EDGE_CURVE ( 'NONE', #12408, #6787, #12876, .T. ) ;
#19673=CARTESIAN_POINT ( 'NONE',  ( 3.118309183252346628, 17.14266753270391774, 1.500000000000000000 ) ) ;
#19688=CIRCLE ( 'NONE', #6270, 37.60050224823048381 ) ;
#19698=( GEOMETRIC_REPRESENTATION_CONTEXT ( 3 ) GLOBAL_UNCERTAINTY_ASSIGNED_CONTEXT ( ( #6438 ) ) GLOBAL_UNIT_ASSIGNED_CONTEXT ( ( #1443, #30274, #6260 ) ) REPRESENTATION_CONTEXT ( 'NONE', 'WORKASPACE' ) );
#19699=VERTEX_POINT ( 'NONE', #18340 ) ;
#19733=CIRCLE ( 'NONE', #14239, 0.6002263538043648428 ) ;
#19742=DIRECTION ( 'NONE',  ( -0.000000000000000000, -0.000000000000000000, -1.000000000000000000 ) ) ;
#19746=CIRCLE ( 'NONE', #1834, 28.20443790117971261 ) ;
#19751=ORIENTED_EDGE ( 'NONE', *, *, #17186, .F. ) ;
#19757=SHAPE_REPRESENTATION_RELATIONSHIP ( 'NONE' , 'NONE' ,  #7129, #574 ) ;
#19758=ORIENTED_EDGE ( 'NONE', *, *, #13033, .F. ) ;
#19766=ORIENTED_EDGE ( 'NONE', *, *, #11998, .F. ) ;
#19779=CARTESIAN_POINT ( 'NONE',  ( 3.118309183252346628, -17.14266753270391774, -1.500000000000000000 ) ) ;
#19791=EDGE_LOOP ( 'NONE', ( #22439, #17766, #14615, #19883, #9047, #5635 ) ) ;
#19793=CLOSED_SHELL ( 'NONE', ( #20245, #13276, #9571, #26526, #10896, #24592, #26151, #2943, #3686, #9327, #20061, #14323, #10495, #16559, #8988, #26907, #16711, #19472, #4444, #8979, #3523, #11490, #29558, #21399, #23652, #23895, #22099, #26770, #28035, #20805, #12244, #8641, #597, #2423, #21740, #22123, #14563, #22318, #23854, #26212, #10713, #9807, #12111, #23247, #5928, #1449, #11112, #30389, #1761, #20276, #18559, #4273, #28847, #18556, #21789, #12835, #7572, #20063, #10505, #6349, #751, #21739, #14362, #13205, #17962, #11941, #23399, #22761, #15846, #18524, #791, #18694, #9746, #24061, #26511, #14487, #21232, #9375, #2924, #21135, #3642, #10666, #25733, #27694, #1383, #1177 ) ) ;
#19802=CIRCLE ( 'NONE', #15244, 2.061368542273053883 ) ;
#19807=ORIENTED_EDGE ( 'NONE', *, *, #22807, .F. ) ;
#19810=VECTOR ( 'NONE', #19993, 1000.000000000000000 ) ;
#19816=EDGE_LOOP ( 'NONE', ( #20979, #17555, #8462, #6615, #13797 ) ) ;
#19819=EDGE_CURVE ( 'NONE', #19699, #2517, #1499, .T. ) ;
#19823=CIRCLE ( 'NONE', #10368, 0.6002263538043648428 ) ;
#19824=AXIS2_PLACEMENT_3D ( 'NONE', #27851, #18636, #1946 ) ;
#19838=CARTESIAN_POINT ( 'NONE',  ( 0.000000000000000000, 0.000000000000000000, -1.500000000000000000 ) ) ;
#19848=DIRECTION ( 'NONE',  ( 1.000000000000000000, 0.000000000000000000, 0.000000000000000000 ) ) ;
#19849=PLANE ( 'NONE',  #29408 ) ;
#19860=DIRECTION ( 'NONE',  ( -0.000000000000000000, 0.000000000000000000, 1.000000000000000000 ) ) ;
#19861=AXIS2_PLACEMENT_3D ( 'NONE', #29182, #15285, #5322 ) ;
#19879=CYLINDRICAL_SURFACE ( 'NONE', #10798, 2.898871837527149165 ) ;
#19883=ORIENTED_EDGE ( 'NONE', *, *, #16264, .F. ) ;
#19892=CIRCLE ( 'NONE', #7942, 32.32717498572574755 ) ;
#19906=CYLINDRICAL_SURFACE ( 'NONE', #22992, 32.32717498572574755 ) ;
#19908=CARTESIAN_POINT ( 'NONE',  ( 30.31220697679117038, 11.23460505553742550, -1.500000000000000000 ) ) ;
#19923=LINE ( 'NONE', #2930, #14053 ) ;
#19926=DIRECTION ( 'NONE',  ( -0.000000000000000000, 0.000000000000000000, 1.000000000000000000 ) ) ;
#19943=CARTESIAN_POINT ( 'NONE',  ( 14.89473990422475680, -17.79239818699420539, -1.500000000000000000 ) ) ;
#19947=DIRECTION ( 'NONE',  ( -0.000000000000000000, -0.000000000000000000, -1.000000000000000000 ) ) ;
#19965=CARTESIAN_POINT ( 'NONE',  ( 8.616279238414451314, -7.781333699927420966, 1.500000000000000000 ) ) ;
#19980=FACE_OUTER_BOUND ( 'NONE', #1523, .T. ) ;
#19993=DIRECTION ( 'NONE',  ( -0.000000000000000000, -0.000000000000000000, -1.000000000000000000 ) ) ;
#20005=DIRECTION ( 'NONE',  ( 1.000000000000000000, 0.000000000000000000, 0.000000000000000000 ) ) ;
#20006=AXIS2_PLACEMENT_3D ( 'NONE', #5381, #12562, #22055 ) ;
#20008=DIRECTION ( 'NONE',  ( -0.000000000000000000, 0.000000000000000000, 1.000000000000000000 ) ) ;
#20021=CARTESIAN_POINT ( 'NONE',  ( 0.000000000000000000, 0.000000000000000000, 1.500000000000000000 ) ) ;
#20035=ORIENTED_EDGE ( 'NONE', *, *, #27893, .F. ) ;
#20048=DIRECTION ( 'NONE',  ( 0.000000000000000000, -0.000000000000000000, -1.000000000000000000 ) ) ;
#20058=CARTESIAN_POINT ( 'NONE',  ( -21.71568325578193637, 0.000000000000000000, -1.500000000000000000 ) ) ;
#20061=ADVANCED_FACE ( 'NONE', ( #27655 ), #4399, .F. ) ;
#20062=EDGE_CURVE ( 'NONE', #29776, #3576, #21305, .T. ) ;
#20063=ADVANCED_FACE ( 'NONE', ( #13630 ), #23260, .F. ) ;
#20066=EDGE_LOOP ( 'NONE', ( #20353, #3830, #3790, #9903 ) ) ;
#20068=VERTEX_POINT ( 'NONE', #10977 ) ;
#20078=ORIENTED_EDGE ( 'NONE', *, *, #15070, .F. ) ;
#20085=CARTESIAN_POINT ( 'NONE',  ( 0.000000000000000000, 0.000000000000000000, 1.500000000000000000 ) ) ;
#20086=CIRCLE ( 'NONE', #28052, 32.32717498572574755 ) ;
#20100=VECTOR ( 'NONE', #9668, 1000.000000000000000 ) ;
#20111=CARTESIAN_POINT ( 'NONE',  ( 28.34828976096171971, -29.18752572968383419, 1.500000000000000000 ) ) ;
#20127=CARTESIAN_POINT ( 'NONE',  ( 0.000000000000000000, 0.000000000000000000, -1.500000000000000000 ) ) ;
#20128=ORIENTED_EDGE ( 'NONE', *, *, #12996, .T. ) ;
#20131=EDGE_CURVE ( 'NONE', #5698, #3354, #855, .T. ) ;
#20149=CARTESIAN_POINT ( 'NONE',  ( -26.83043119477639493, -8.695877139419037505, 1.500000000000000000 ) ) ;
#20174=CARTESIAN_POINT ( 'NONE',  ( -19.54426622602688113, 37.07991288358297055, 1.499999999999999778 ) ) ;
#20176=EDGE_LOOP ( 'NONE', ( #26492, #1582, #18105, #8932 ) ) ;
#20195=ORIENTED_EDGE ( 'NONE', *, *, #27534, .F. ) ;
#20198=CARTESIAN_POINT ( 'NONE',  ( -8.419710366748644148, 7.777014463793872956, -1.500000000000000000 ) ) ;
#20205=LINE ( 'NONE', #23002, #27492 ) ;
#20227=VECTOR ( 'NONE', #25105, 1000.000000000000000 ) ;
#20230=EDGE_LOOP ( 'NONE', ( #30587, #204 ) ) ;
#20232=EDGE_CURVE ( 'NONE', #20433, #1352, #21754, .T. ) ;
#20233=ORIENTED_EDGE ( 'NONE', *, *, #22241, .T. ) ;
#20245=ADVANCED_FACE ( 'NONE', ( #28263 ), #23560, .T. ) ;
#20252=AXIS2_PLACEMENT_3D ( 'NONE', #6631, #27550, #22854 ) ;
#20274=AXIS2_PLACEMENT_3D ( 'NONE', #3531, #5554, #22537 ) ;
#20276=ADVANCED_FACE ( 'NONE', ( #19980 ), #15283, .F. ) ;
#20284=EDGE_CURVE ( 'NONE', #16393, #6819, #22158, .T. ) ;
#20287=DIRECTION ( 'NONE',  ( -0.000000000000000000, -0.000000000000000000, -1.000000000000000000 ) ) ;
#20289=AXIS2_PLACEMENT_3D ( 'NONE', #29824, #7827, #26698 ) ;
#20295=DIRECTION ( 'NONE',  ( 0.000000000000000000, -0.000000000000000000, -1.000000000000000000 ) ) ;
#20315=CARTESIAN_POINT ( 'NONE',  ( 2.599508007902112006, 14.29059753516471964, 1.500000000000000000 ) ) ;
#20318=FACE_OUTER_BOUND ( 'NONE', #20737, .T. ) ;
#20325=AXIS2_PLACEMENT_3D ( 'NONE', #4098, #13764, #15791 ) ;
#20345=CARTESIAN_POINT ( 'NONE',  ( 26.44644203219471379, 9.801837641955973623, -1.500000000000000000 ) ) ;
#20353=ORIENTED_EDGE ( 'NONE', *, *, #10703, .F. ) ;
#20361=CARTESIAN_POINT ( 'NONE',  ( 14.41708049311143469, -17.22181377297010130, 1.500000000000000000 ) ) ;
#20368=FACE_OUTER_BOUND ( 'NONE', #1611, .T. ) ;
#20370=DIRECTION ( 'NONE',  ( -0.000000000000000000, 0.000000000000000000, 1.000000000000000000 ) ) ;
#20393=CIRCLE ( 'NONE', #14910, 28.20443790117963800 ) ;
#20402=ORIENTED_EDGE ( 'NONE', *, *, #13579, .F. ) ;
#20409=FACE_BOUND ( 'NONE', #10338, .T. ) ;
#20433=VERTEX_POINT ( 'NONE', #3234 ) ;
#20436=VERTEX_POINT ( 'NONE', #16166 ) ;
#20452=ORIENTED_EDGE ( 'NONE', *, *, #28416, .F. ) ;
#20454=CARTESIAN_POINT ( 'NONE',  ( 28.79137815760242702, -9.331429872129930914, 1.500000000000000000 ) ) ;
#20459=DIRECTION ( 'NONE',  ( 1.000000000000000000, 0.000000000000000000, 0.000000000000000000 ) ) ;
#20469=EDGE_CURVE ( 'NONE', #15101, #14162, #7262, .T. ) ;
#20479=DIRECTION ( 'NONE',  ( -0.000000000000000000, -0.000000000000000000, -1.000000000000000000 ) ) ;
#20496=ORIENTED_EDGE ( 'NONE', *, *, #4074, .T. ) ;
#20502=CARTESIAN_POINT ( 'NONE',  ( -14.89473990422384198, 17.79239818699320708, -1.500000000000000000 ) ) ;
#20506=CARTESIAN_POINT ( 'NONE',  ( -1.073881485057887497, 0.9711784013062738641, 1.500000000000000000 ) ) ;
#20527=CARTESIAN_POINT ( 'NONE',  ( -4.163336342344337027E-14, 1.387778780781445676E-14, 1.500000000000000000 ) ) ;
#20530=CIRCLE ( 'NONE', #26962, 0.7441270634457163302 ) ;
#20539=ORIENTED_EDGE ( 'NONE', *, *, #27685, .T. ) ;
#20544=LINE ( 'NONE', #13545, #21493 ) ;
#20571=ORIENTED_EDGE ( 'NONE', *, *, #25937, .T. ) ;
#20573=CARTESIAN_POINT ( 'NONE',  ( 0.000000000000000000, 5.590849009245238754, 1.500000000000000000 ) ) ;
#20609=DIRECTION ( 'NONE',  ( 0.000000000000000000, -0.000000000000000000, -1.000000000000000000 ) ) ;
#20617=EDGE_CURVE ( 'NONE', #21731, #14945, #12573, .T. ) ;
#20626=DIRECTION ( 'NONE',  ( 1.000000000000000000, 0.000000000000000000, 0.000000000000000000 ) ) ;
#20644=VERTEX_POINT ( 'NONE', #14194 ) ;
#20648=CIRCLE ( 'NONE', #24115, 2.898871837527149609 ) ;
#20676=EDGE_LOOP ( 'NONE', ( #9748, #1158, #26324, #22167, #7680, #2042 ) ) ;
#20687=CIRCLE ( 'NONE', #17692, 32.32717498572581860 ) ;
#20691=ORIENTED_EDGE ( 'NONE', *, *, #20971, .T. ) ;
#20696=AXIS2_PLACEMENT_3D ( 'NONE', #6283, #22818, #15961 ) ;
#20717=EDGE_LOOP ( 'NONE', ( #17905, #3040, #9675, #1411 ) ) ;
#20737=EDGE_LOOP ( 'NONE', ( #16175, #27039, #11679, #4393 ) ) ;
#20739=VECTOR ( 'NONE', #23896, 1000.000000000000000 ) ;
#20740=DIRECTION ( 'NONE',  ( -1.000000000000000000, 0.000000000000000000, 0.000000000000000000 ) ) ;
#20756=ORIENTED_EDGE ( 'NONE', *, *, #3465, .T. ) ;
#20766=AXIS2_PLACEMENT_3D ( 'NONE', #26175, #282, #12147 ) ;
#20773=EDGE_LOOP ( 'NONE', ( #4836, #18286, #20452, #248 ) ) ;
#20785=EDGE_LOOP ( 'NONE', ( #13576, #4302, #13578, #16953 ) ) ;
#20795=AXIS2_PLACEMENT_3D ( 'NONE', #20085, #15396, #15227 ) ;
#20796=DIRECTION ( 'NONE',  ( 0.000000000000000000, -0.000000000000000000, -1.000000000000000000 ) ) ;
#20805=ADVANCED_FACE ( 'NONE', ( #4232 ), #16238, .F. ) ;
#20822=CARTESIAN_POINT ( 'NONE',  ( -32.32717498572578307, -1.387778780781445676E-14, 1.500000000000000000 ) ) ;
#20849=LINE ( 'NONE', #30375, #11563 ) ;
#20854=CARTESIAN_POINT ( 'NONE',  ( -32.32717498572578307, -1.387778780781445676E-14, -1.500000000000000000 ) ) ;
#20871=ORIENTED_EDGE ( 'NONE', *, *, #12317, .F. ) ;
#20890=FACE_BOUND ( 'NONE', #4246, .T. ) ;
#20894=EDGE_CURVE ( 'NONE', #12321, #25145, #1416, .T. ) ;
#20898=ORIENTED_EDGE ( 'NONE', *, *, #21996, .F. ) ;
#20932=DIRECTION ( 'NONE',  ( 0.4495526574063634095, -0.8932538319083086487, 0.000000000000000000 ) ) ;
#20938=VERTEX_POINT ( 'NONE', #29640 ) ;
#20941=DIRECTION ( 'NONE',  ( 1.000000000000000000, 0.000000000000000000, 0.000000000000000000 ) ) ;
#20951=LINE ( 'NONE', #18640, #15857 ) ;
#20961=CARTESIAN_POINT ( 'NONE',  ( -14.89473990422384198, 17.79239818699320708, 1.500000000000000000 ) ) ;
#20971=EDGE_CURVE ( 'NONE', #21504, #18859, #21878, .T. ) ;
#20979=ORIENTED_EDGE ( 'NONE', *, *, #7849, .F. ) ;
#20986=VERTEX_POINT ( 'NONE', #29490 ) ;
#20988=DIRECTION ( 'NONE',  ( 0.6707505147970024284, 0.7416830501633134842, 0.000000000000000000 ) ) ;
#20990=VERTEX_POINT ( 'NONE', #15269 ) ;
#21014=DIRECTION ( 'NONE',  ( 1.000000000000000000, 0.000000000000000000, 0.000000000000000000 ) ) ;
#21020=CARTESIAN_POINT ( 'NONE',  ( -15.57266529552203416, 38.96488032230103471, -1.500000000000000000 ) ) ;
#21026=DIRECTION ( 'NONE',  ( 0.000000000000000000, -0.000000000000000000, -1.000000000000000000 ) ) ;
#21029=VERTEX_POINT ( 'NONE', #25717 ) ;
#21036=VECTOR ( 'NONE', #20287, 1000.000000000000000 ) ;
#21056=ORIENTED_EDGE ( 'NONE', *, *, #24795, .F. ) ;
#21076=FACE_OUTER_BOUND ( 'NONE', #7001, .T. ) ;
#21077=VERTEX_POINT ( 'NONE', #30405 ) ;
#21090=ORIENTED_EDGE ( 'NONE', *, *, #23526, .F. ) ;
#21092=CARTESIAN_POINT ( 'NONE',  ( -4.163336342344337027E-14, -1.387778780781445676E-14, 1.500000000000000000 ) ) ;
#21108=CARTESIAN_POINT ( 'NONE',  ( 23.17581250239727808, -34.50630206824671831, 1.499999999999999778 ) ) ;
#21110=LINE ( 'NONE', #1800, #10797 ) ;
#21124=ORIENTED_EDGE ( 'NONE', *, *, #7435, .F. ) ;
#21134=PLANE ( 'NONE',  #13845 ) ;
#21135=ADVANCED_FACE ( 'NONE', ( #7471 ), #30850, .T. ) ;
#21157=VERTEX_POINT ( 'NONE', #19315 ) ;
#21161=ORIENTED_EDGE ( 'NONE', *, *, #63, .T. ) ;
#21167=EDGE_CURVE ( 'NONE', #22347, #22720, #12300, .T. ) ;
#21194=EDGE_CURVE ( 'NONE', #14945, #16254, #1879, .T. ) ;
#21220=DIRECTION ( 'NONE',  ( 1.000000000000000000, 0.000000000000000000, 0.000000000000000000 ) ) ;
#21225=CARTESIAN_POINT ( 'NONE',  ( 26.36764545593179676, 31.31467416275351923, 1.500000000000000000 ) ) ;
#21232=ADVANCED_FACE ( 'NONE', ( #29919 ), #12929, .T. ) ;
#21249=VECTOR ( 'NONE', #29180, 1000.000000000000000 ) ;
#21255=AXIS2_PLACEMENT_3D ( 'NONE', #20454, #29973, #11242 ) ;
#21258=ORIENTED_EDGE ( 'NONE', *, *, #30198, .F. ) ;
#21296=AXIS2_PLACEMENT_3D ( 'NONE', #10550, #20370, #13520 ) ;
#21305=CIRCLE ( 'NONE', #29296, 1.447898107987198646 ) ;
#21308=CARTESIAN_POINT ( 'NONE',  ( -26.36764545593177544, 31.31467416275353344, 1.500000000000000000 ) ) ;
#21310=DIRECTION ( 'NONE',  ( -0.000000000000000000, -0.000000000000000000, -1.000000000000000000 ) ) ;
#21319=AXIS2_PLACEMENT_3D ( 'NONE', #17457, #26657, #2795 ) ;
#21324=ORIENTED_EDGE ( 'NONE', *, *, #14766, .T. ) ;
#21336=EDGE_LOOP ( 'NONE', ( #26092, #2003, #23189, #26884 ) ) ;
#21337=CARTESIAN_POINT ( 'NONE',  ( 3.221450758838616757, -1.621276839356792454, 1.500000000000000000 ) ) ;
#21371=CARTESIAN_POINT ( 'NONE',  ( -4.163336342344337027E-14, 1.387778780781445676E-14, 1.500000000000000000 ) ) ;
#21381=EDGE_LOOP ( 'NONE', ( #12735, #9456, #3846, #17282 ) ) ;
#21398=DIRECTION ( 'NONE',  ( -0.000000000000000000, 0.000000000000000000, 1.000000000000000000 ) ) ;
#21399=ADVANCED_FACE ( 'NONE', ( #1675 ), #21134, .T. ) ;
#21402=ORIENTED_EDGE ( 'NONE', *, *, #20971, .F. ) ;
#21416=CIRCLE ( 'NONE', #1017, 14.52510309069108807 ) ;
#21431=ORIENTED_EDGE ( 'NONE', *, *, #27895, .F. ) ;
#21493=VECTOR ( 'NONE', #20988, 1000.000000000000000 ) ;
#21504=VERTEX_POINT ( 'NONE', #15871 ) ;
#21529=AXIS2_PLACEMENT_3D ( 'NONE', #10006, #26537, #21684 ) ;
#21532=VECTOR ( 'NONE', #9597, 1000.000000000000114 ) ;
#21545=CARTESIAN_POINT ( 'NONE',  ( -14.36006998371493637, -17.26937953831884442, 1.500000000000000000 ) ) ;
#21549=EDGE_LOOP ( 'NONE', ( #27612, #30834, #8963, #7508 ) ) ;
#21560=ORIENTED_EDGE ( 'NONE', *, *, #28037, .T. ) ;
#21565=DIRECTION ( 'NONE',  ( 1.000000000000000000, 0.000000000000000000, 0.000000000000000000 ) ) ;
#21566=ORIENTED_EDGE ( 'NONE', *, *, #16891, .T. ) ;
#21582=EDGE_CURVE ( 'NONE', #3169, #15101, #24297, .T. ) ;
#21591=DIRECTION ( 'NONE',  ( -0.6707505147970012072, 0.7416830501633145944, 0.000000000000000000 ) ) ;
#21594=ORIENTED_EDGE ( 'NONE', *, *, #8039, .T. ) ;
#21597=CARTESIAN_POINT ( 'NONE',  ( -8.860628911697515875, 8.184276679720483116, 1.500000000000000000 ) ) ;
#21624=DIRECTION ( 'NONE',  ( 1.000000000000000000, 0.000000000000000000, 0.000000000000000000 ) ) ;
#21626=VECTOR ( 'NONE', #26994, 1000.000000000000000 ) ;
#21641=DIRECTION ( 'NONE',  ( 0.000000000000000000, -0.000000000000000000, -1.000000000000000000 ) ) ;
#21650=VERTEX_POINT ( 'NONE', #29102 ) ;
#21683=FACE_OUTER_BOUND ( 'NONE', #21549, .T. ) ;
#21684=DIRECTION ( 'NONE',  ( 0.6707505147970089787, 0.7416830501633076000, 0.000000000000000000 ) ) ;
#21691=DIRECTION ( 'NONE',  ( -0.000000000000000000, 0.000000000000000000, 1.000000000000000000 ) ) ;
#21693=AXIS2_PLACEMENT_3D ( 'NONE', #30478, #16297, #2090 ) ;
#21699=CARTESIAN_POINT ( 'NONE',  ( -14.83584055149731817, -17.84153987719691514, -1.500000000000000000 ) ) ;
#21715=EDGE_LOOP ( 'NONE', ( #25616, #29646, #12960, #12374 ) ) ;
#21717=VERTEX_POINT ( 'NONE', #3359 ) ;
#21725=VERTEX_POINT ( 'NONE', #12892 ) ;
#21731=VERTEX_POINT ( 'NONE', #12579 ) ;
#21739=ADVANCED_FACE ( 'NONE', ( #24414 ), #27221, .F. ) ;
#21740=ADVANCED_FACE ( 'NONE', ( #24564 ), #12730, .F. ) ;
#21748=EDGE_CURVE ( 'NONE', #14669, #10421, #19823, .T. ) ;
#21754=CIRCLE ( 'NONE', #22266, 0.7441270634456955690 ) ;
#21768=EDGE_CURVE ( 'NONE', #6600, #27382, #21822, .T. ) ;
#21769=DIRECTION ( 'NONE',  ( -0.000000000000000000, -0.000000000000000000, -1.000000000000000000 ) ) ;
#21782=CARTESIAN_POINT ( 'NONE',  ( -14.41708049311053053, 17.22181377296911720, 1.500000000000000000 ) ) ;
#21789=ADVANCED_FACE ( 'NONE', ( #27391 ), #1028, .F. ) ;
#21795=CIRCLE ( 'NONE', #14299, 21.71568325578193637 ) ;
#21807=ORIENTED_EDGE ( 'NONE', *, *, #13563, .F. ) ;
#21822=CIRCLE ( 'NONE', #2414, 14.52510309069105965 ) ;
#21843=ORIENTED_EDGE ( 'NONE', *, *, #17585, .T. ) ;
#21854=EDGE_CURVE ( 'NONE', #19078, #7329, #18633, .T. ) ;
#21862=CIRCLE ( 'NONE', #13897, 10.00000000000000000 ) ;
#21878=( BOUNDED_CURVE ( )  B_SPLINE_CURVE ( 3, ( #27002, #5629, #8590, #15123 ),
 .UNSPECIFIED., .F., .T. ) 
 B_SPLINE_CURVE_WITH_KNOTS ( ( 4, 4 ),
 ( 5.540737561276206868, 5.872433067142492469 ),
 .UNSPECIFIED. ) 
 CURVE ( )  GEOMETRIC_REPRESENTATION_ITEM ( )  RATIONAL_B_SPLINE_CURVE ( ( 1.000000000000000000, 0.9908525036704132205, 0.9908525036704132205, 1.000000000000000000 ) ) 
 REPRESENTATION_ITEM ( '' )  );
#21883=AXIS2_PLACEMENT_3D ( 'NONE', #81, #7246, #21591 ) ;
#21884=ORIENTED_EDGE ( 'NONE', *, *, #2235, .T. ) ;
#21894=DIRECTION ( 'NONE',  ( -0.4495526574063634095, 0.8932538319083086487, 0.000000000000000000 ) ) ;
#21907=DIRECTION ( 'NONE',  ( -0.000000000000000000, -0.000000000000000000, -1.000000000000000000 ) ) ;
#21909=LINE ( 'NONE', #5848, #121 ) ;
#21925=DIRECTION ( 'NONE',  ( -0.000000000000000000, -0.000000000000000000, -1.000000000000000000 ) ) ;
#21927=ORIENTED_EDGE ( 'NONE', *, *, #16972, .T. ) ;
#21929=DIRECTION ( 'NONE',  ( -0.000000000000000000, -0.000000000000000000, -1.000000000000000000 ) ) ;
#21936=ORIENTED_EDGE ( 'NONE', *, *, #20894, .F. ) ;
#21948=CARTESIAN_POINT ( 'NONE',  ( -26.36764545593177544, -31.31467416275353344, 1.500000000000000000 ) ) ;
#21949=ORIENTED_EDGE ( 'NONE', *, *, #11661, .T. ) ;
#21971=ORIENTED_EDGE ( 'NONE', *, *, #16253, .T. ) ;
#21972=EDGE_CURVE ( 'NONE', #8400, #7329, #8397, .T. ) ;
#21986=ORIENTED_EDGE ( 'NONE', *, *, #4768, .T. ) ;
#21996=EDGE_CURVE ( 'NONE', #20433, #15822, #29316, .T. ) ;
#22024=VERTEX_POINT ( 'NONE', #24995 ) ;
#22030=CIRCLE ( 'NONE', #9594, 20.32284676574536064 ) ;
#22032=ORIENTED_EDGE ( 'NONE', *, *, #5727, .T. ) ;
#22048=FACE_OUTER_BOUND ( 'NONE', #10717, .T. ) ;
#22054=( BOUNDED_CURVE ( )  B_SPLINE_CURVE ( 3, ( #10668, #20174, #4113, #30011 ),
 .UNSPECIFIED., .F., .F. ) 
 B_SPLINE_CURVE_WITH_KNOTS ( ( 4, 4 ),
 ( 0.4107522400370940407, 0.7424477459033789195 ),
 .UNSPECIFIED. ) 
 CURVE ( )  GEOMETRIC_REPRESENTATION_ITEM ( )  RATIONAL_B_SPLINE_CURVE ( ( 1.000000000000000000, 0.9908525036704132205, 0.9908525036704132205, 1.000000000000000000 ) ) 
 REPRESENTATION_ITEM ( '' )  );
#22055=DIRECTION ( 'NONE',  ( -1.000000000000000000, 0.000000000000000000, 0.000000000000000000 ) ) ;
#22070=DIRECTION ( 'NONE',  ( -0.000000000000000000, -0.000000000000000000, -1.000000000000000000 ) ) ;
#22074=CARTESIAN_POINT ( 'NONE',  ( 24.03057240117691862, 26.57182937991349903, 1.500000000000000000 ) ) ;
#22081=DIRECTION ( 'NONE',  ( 1.000000000000000000, 0.000000000000000000, 0.000000000000000000 ) ) ;
#22099=ADVANCED_FACE ( 'NONE', ( #3485 ), #26890, .F. ) ;
#22105=EDGE_LOOP ( 'NONE', ( #13491, #27833, #21402, #25037 ) ) ;
#22116=CARTESIAN_POINT ( 'NONE',  ( -19.54426622602688468, 37.07991288358297055, -1.499999999999999778 ) ) ;
#22123=ADVANCED_FACE ( 'NONE', ( #518 ), #24528, .T. ) ;
#22127=DIRECTION ( 'NONE',  ( -0.000000000000000000, 0.000000000000000000, 1.000000000000000000 ) ) ;
#22158=LINE ( 'NONE', #17168, #21249 ) ;
#22167=ORIENTED_EDGE ( 'NONE', *, *, #23049, .F. ) ;
#22191=CARTESIAN_POINT ( 'NONE',  ( -3.515970705488605130, 17.06554576617236307, -1.500000000000000000 ) ) ;
#22194=AXIS2_PLACEMENT_3D ( 'NONE', #12901, #6323, #15836 ) ;
#22199=FACE_OUTER_BOUND ( 'NONE', #29086, .T. ) ;
#22200=EDGE_LOOP ( 'NONE', ( #10387, #20035, #11856, #25032 ) ) ;
#22206=VECTOR ( 'NONE', #5650, 1000.000000000000000 ) ;
#22217=ORIENTED_EDGE ( 'NONE', *, *, #16064, .T. ) ;
#22220=VECTOR ( 'NONE', #21310, 1000.000000000000000 ) ;
#22240=CARTESIAN_POINT ( 'NONE',  ( 0.000000000000000000, 0.000000000000000000, -1.500000000000000000 ) ) ;
#22241=EDGE_CURVE ( 'NONE', #6747, #3010, #23314, .T. ) ;
#22245=EDGE_LOOP ( 'NONE', ( #16113, #11666, #26544, #11469 ) ) ;
#22248=EDGE_LOOP ( 'NONE', ( #29890, #15777, #21884, #13332 ) ) ;
#22253=VECTOR ( 'NONE', #29270, 1000.000000000000000 ) ;
#22254=( NAMED_UNIT ( * ) SI_UNIT ( $, .STERADIAN. ) SOLID_ANGLE_UNIT ( ) );
#22255=AXIS2_PLACEMENT_3D ( 'NONE', #21545, #17027, #180 ) ;
#22266=AXIS2_PLACEMENT_3D ( 'NONE', #30745, #9232, #16709 ) ;
#22270=LINE ( 'NONE', #15715, #2655 ) ;
#22271=AXIS2_PLACEMENT_3D ( 'NONE', #29785, #18080, #6222 ) ;
#22285=FACE_OUTER_BOUND ( 'NONE', #30387, .T. ) ;
#22318=ADVANCED_FACE ( 'NONE', ( #24490 ), #17322, .F. ) ;
#22321=EDGE_CURVE ( 'NONE', #21077, #8486, #12658, .T. ) ;
#22323=CARTESIAN_POINT ( 'NONE',  ( 8.860628911697515875, 8.184276679720483116, -1.500000000000000000 ) ) ;
#22331=CYLINDRICAL_SURFACE ( 'NONE', #1394, 2.898871837527151829 ) ;
#22344=ORIENTED_EDGE ( 'NONE', *, *, #4019, .T. ) ;
#22347=VERTEX_POINT ( 'NONE', #28825 ) ;
#22373=CARTESIAN_POINT ( 'NONE',  ( -30.31220697679117393, 11.23460505553742550, 1.500000000000000000 ) ) ;
#22382=CIRCLE ( 'NONE', #9911, 0.7441270634457163302 ) ;
#22392=DIRECTION ( 'NONE',  ( 1.000000000000000000, 0.000000000000000000, 0.000000000000000000 ) ) ;
#22393=DIRECTION ( 'NONE',  ( -0.000000000000000000, -0.000000000000000000, -1.000000000000000000 ) ) ;
#22417=ORIENTED_EDGE ( 'NONE', *, *, #6720, .F. ) ;
#22430=CYLINDRICAL_SURFACE ( 'NONE', #13766, 2.061368542273053883 ) ;
#22433=FACE_BOUND ( 'NONE', #19791, .T. ) ;
#22439=ORIENTED_EDGE ( 'NONE', *, *, #9612, .T. ) ;
#22440=CARTESIAN_POINT ( 'NONE',  ( 0.000000000000000000, 0.000000000000000000, -1.500000000000000000 ) ) ;
#22443=ORIENTED_EDGE ( 'NONE', *, *, #2711, .F. ) ;
#22457=DIRECTION ( 'NONE',  ( -0.000000000000000000, -0.000000000000000000, -1.000000000000000000 ) ) ;
#22461=CIRCLE ( 'NONE', #18985, 23.20393738267342698 ) ;
#22479=ORIENTED_EDGE ( 'NONE', *, *, #27895, .T. ) ;
#22496=EDGE_CURVE ( 'NONE', #3349, #16393, #9894, .T. ) ;
#22524=EDGE_LOOP ( 'NONE', ( #11097, #23684, #17577, #28601 ) ) ;
#22532=EDGE_CURVE ( 'NONE', #4573, #27291, #18200, .T. ) ;
#22534=LINE ( 'NONE', #27542, #1884 ) ;
#22537=DIRECTION ( 'NONE',  ( -1.000000000000000000, 0.000000000000000000, 0.000000000000000000 ) ) ;
#22550=DIRECTION ( 'NONE',  ( -1.000000000000000000, 0.000000000000000000, 0.000000000000000000 ) ) ;
#22551=EDGE_LOOP ( 'NONE', ( #3115, #26591, #27216, #10104 ) ) ;
#22576=CARTESIAN_POINT ( 'NONE',  ( 22.95669091611928181, 27.54300778121952575, 1.500000000000000000 ) ) ;
#22612=EDGE_LOOP ( 'NONE', ( #9801, #24515, #18456, #17041 ) ) ;
#22633=FACE_OUTER_BOUND ( 'NONE', #16221, .T. ) ;
#22647=CARTESIAN_POINT ( 'NONE',  ( 1.073881485057758711, 0.9711784013061475207, 1.500000000000000000 ) ) ;
#22664=EDGE_LOOP ( 'NONE', ( #27807, #3893, #23420, #21560 ) ) ;
#22670=DIRECTION ( 'NONE',  ( 1.000000000000000000, 4.440892098500625373E-15, 0.000000000000000000 ) ) ;
#22678=DIRECTION ( 'NONE',  ( -0.6707505147970128645, -0.7416830501633041584, 0.000000000000000000 ) ) ;
#22683=AXIS2_PLACEMENT_3D ( 'NONE', #16722, #21398, #24037 ) ;
#22687=EDGE_CURVE ( 'NONE', #6050, #2551, #25349, .T. ) ;
#22688=LINE ( 'NONE', #1341, #22253 ) ;
#22693=EDGE_CURVE ( 'NONE', #6050, #12408, #18361, .T. ) ;
#22712=ORIENTED_EDGE ( 'NONE', *, *, #265, .F. ) ;
#22720=VERTEX_POINT ( 'NONE', #4003 ) ;
#22722=CARTESIAN_POINT ( 'NONE',  ( -6.414842543015754295, 17.06554576617236307, 1.500000000000000000 ) ) ;
#22726=EDGE_CURVE ( 'NONE', #9342, #22982, #28845, .T. ) ;
#22730=EDGE_CURVE ( 'NONE', #19427, #3343, #18511, .T. ) ;
#22748=CARTESIAN_POINT ( 'NONE',  ( -9.675133109038686285, -8.168544852422948921, 1.500000000000000000 ) ) ;
#22754=LINE ( 'NONE', #29636, #20227 ) ;
#22761=ADVANCED_FACE ( 'NONE', ( #26282 ), #16765, .F. ) ;
#22768=CARTESIAN_POINT ( 'NONE',  ( -28.34828976096172681, 29.18752572968383419, 1.500000000000000000 ) ) ;
#22777=ORIENTED_EDGE ( 'NONE', *, *, #19819, .T. ) ;
#22778=VECTOR ( 'NONE', #7987, 1000.000000000000000 ) ;
#22794=DIRECTION ( 'NONE',  ( -0.000000000000000000, 0.000000000000000000, 1.000000000000000000 ) ) ;
#22798=FACE_OUTER_BOUND ( 'NONE', #8446, .T. ) ;
#22807=EDGE_CURVE ( 'NONE', #24290, #9920, #1473, .T. ) ;
#22818=DIRECTION ( 'NONE',  ( 0.000000000000000000, -0.000000000000000000, -1.000000000000000000 ) ) ;
#22821=CIRCLE ( 'NONE', #27824, 2.898871837527151385 ) ;
#22839=ORIENTED_EDGE ( 'NONE', *, *, #8049, .T. ) ;
#22850=ORIENTED_EDGE ( 'NONE', *, *, #22241, .F. ) ;
#22854=DIRECTION ( 'NONE',  ( 1.000000000000000000, 0.000000000000000000, 0.000000000000000000 ) ) ;
#22885=VERTEX_POINT ( 'NONE', #20345 ) ;
#22894=DIRECTION ( 'NONE',  ( -0.000000000000000000, 0.000000000000000000, 1.000000000000000000 ) ) ;
#22926=CARTESIAN_POINT ( 'NONE',  ( 8.757878075398934925, -7.394122547431893011, 1.500000000000000000 ) ) ;
#22931=DIRECTION ( 'NONE',  ( 1.000000000000000000, 2.396195514597832977E-15, 0.000000000000000000 ) ) ;
#22939=EDGE_CURVE ( 'NONE', #28942, #26950, #29862, .T. ) ;
#22950=DIRECTION ( 'NONE',  ( -0.000000000000000000, 0.000000000000000000, 1.000000000000000000 ) ) ;
#22968=DIRECTION ( 'NONE',  ( -1.000000000000000000, 0.000000000000000000, 0.000000000000000000 ) ) ;
#22982=VERTEX_POINT ( 'NONE', #13610 ) ;
#22987=LINE ( 'NONE', #29563, #7374 ) ;
#22992=AXIS2_PLACEMENT_3D ( 'NONE', #10686, #22393, #17413 ) ;
#22994=FACE_OUTER_BOUND ( 'NONE', #12433, .T. ) ;
#23002=CARTESIAN_POINT ( 'NONE',  ( 16.65122935894595813, 13.93942108199718888, 1.500000000000000000 ) ) ;
#23025=ORIENTED_EDGE ( 'NONE', *, *, #251, .F. ) ;
#23036=CARTESIAN_POINT ( 'NONE',  ( 0.000000000000000000, 0.000000000000000000, 1.500000000000000000 ) ) ;
#23037=EDGE_LOOP ( 'NONE', ( #4342, #8189, #6842, #24125 ) ) ;
#23047=ORIENTED_EDGE ( 'NONE', *, *, #15854, .T. ) ;
#23049=EDGE_CURVE ( 'NONE', #26988, #10311, #30359, .T. ) ;
#23063=CARTESIAN_POINT ( 'NONE',  ( 9.216505592218814158, -7.781333699927420966, 1.500000000000000000 ) ) ;
#23081=DIRECTION ( 'NONE',  ( -0.000000000000000000, -0.000000000000000000, -1.000000000000000000 ) ) ;
#23103=LINE ( 'NONE', #29992, #12529 ) ;
#23107=CARTESIAN_POINT ( 'NONE',  ( 28.37932450449293853, 10.51822134874671022, 1.500000000000000000 ) ) ;
#23112=DIRECTION ( 'NONE',  ( -1.000000000000000000, 0.000000000000000000, 0.000000000000000000 ) ) ;
#23136=CARTESIAN_POINT ( 'NONE',  ( -14.41708049311053053, 17.22181377296911720, -1.500000000000000000 ) ) ;
#23177=DIRECTION ( 'NONE',  ( 0.6707505147970127535, 0.7416830501633041584, 0.000000000000000000 ) ) ;
#23189=ORIENTED_EDGE ( 'NONE', *, *, #7075, .T. ) ;
#23195=VECTOR ( 'NONE', #9662, 1000.000000000000000 ) ;
#23198=ORIENTED_EDGE ( 'NONE', *, *, #6167, .F. ) ;
#23201=ORIENTED_EDGE ( 'NONE', *, *, #26926, .F. ) ;
#23228=ORIENTED_EDGE ( 'NONE', *, *, #6720, .T. ) ;
#23234=LINE ( 'NONE', #7025, #16118 ) ;
#23247=ADVANCED_FACE ( 'NONE', ( #24947 ), #12953, .F. ) ;
#23249=EDGE_CURVE ( 'NONE', #10311, #15107, #17310, .T. ) ;
#23260=CYLINDRICAL_SURFACE ( 'NONE', #10371, 2.061368542273053883 ) ;
#23261=VECTOR ( 'NONE', #13432, 1000.000000000000114 ) ;
#23273=DIRECTION ( 'NONE',  ( -0.000000000000000000, -0.000000000000000000, -1.000000000000000000 ) ) ;
#23303=CIRCLE ( 'NONE', #18339, 2.061368542273053883 ) ;
#23314=CIRCLE ( 'NONE', #9871, 21.71568325578202163 ) ;
#23317=LINE ( 'NONE', #20822, #17510 ) ;
#23336=LINE ( 'NONE', #24796, #15706 ) ;
#23343=DIRECTION ( 'NONE',  ( -0.000000000000000000, -0.000000000000000000, -1.000000000000000000 ) ) ;
#23349=DIRECTION ( 'NONE',  ( -0.000000000000000000, -0.000000000000000000, -1.000000000000000000 ) ) ;
#23359=AXIS2_PLACEMENT_3D ( 'NONE', #28479, #12101, #12412 ) ;
#23361=VERTEX_POINT ( 'NONE', #14628 ) ;
#23375=ORIENTED_EDGE ( 'NONE', *, *, #13952, .F. ) ;
#23380=ORIENTED_EDGE ( 'NONE', *, *, #7140, .T. ) ;
#23381=CARTESIAN_POINT ( 'NONE',  ( 1.073881485057738949, -0.9711784013061123266, 1.500000000000000000 ) ) ;
#23382=DIRECTION ( 'NONE',  ( -0.000000000000000000, 0.000000000000000000, 1.000000000000000000 ) ) ;
#23399=ADVANCED_FACE ( 'NONE', ( #14154 ), #28828, .F. ) ;
#23410=CARTESIAN_POINT ( 'NONE',  ( -4.163336342344337027E-14, -1.387778780781445676E-14, -1.500000000000000000 ) ) ;
#23411=EDGE_CURVE ( 'NONE', #18893, #8846, #14439, .T. ) ;
#23415=LINE ( 'NONE', #13915, #18983 ) ;
#23420=ORIENTED_EDGE ( 'NONE', *, *, #13002, .T. ) ;
#23426=LINE ( 'NONE', #2843, #20739 ) ;
#23430=CARTESIAN_POINT ( 'NONE',  ( -3.515970705488605130, 17.06554576617236307, 1.500000000000000000 ) ) ;
#23433=EDGE_CURVE ( 'NONE', #7456, #4466, #1490, .T. ) ;
#23449=VERTEX_POINT ( 'NONE', #15820 ) ;
#23451=CARTESIAN_POINT ( 'NONE',  ( 3.118309183252346628, 17.14266753270391774, 1.500000000000000000 ) ) ;
#23453=CARTESIAN_POINT ( 'NONE',  ( 19.54426622602687758, -37.07991288358297055, 1.499999999999999778 ) ) ;
#23466=ORIENTED_EDGE ( 'NONE', *, *, #3100, .F. ) ;
#23476=EDGE_CURVE ( 'NONE', #14300, #6600, #14079, .T. ) ;
#23492=CIRCLE ( 'NONE', #6591, 2.898871837527149609 ) ;
#23515=CARTESIAN_POINT ( 'NONE',  ( -16.69721919944057831, 13.88429941593312122, -1.500000000000000000 ) ) ;
#23520=DIRECTION ( 'NONE',  ( -0.000000000000000000, 0.000000000000000000, 1.000000000000000000 ) ) ;
#23526=EDGE_CURVE ( 'NONE', #16767, #3169, #10453, .T. ) ;
#23530=FACE_BOUND ( 'NONE', #6925, .T. ) ;
#23532=VECTOR ( 'NONE', #20932, 1000.000000000000000 ) ;
#23553=DIRECTION ( 'NONE',  ( -0.000000000000000000, 0.000000000000000000, 1.000000000000000000 ) ) ;
#23556=EDGE_LOOP ( 'NONE', ( #7925, #21324, #17596, #28894 ) ) ;
#23560=CYLINDRICAL_SURFACE ( 'NONE', #13795, 21.71568325578193637 ) ;
#23568=AXIS2_PLACEMENT_3D ( 'NONE', #26033, #25585, #11544 ) ;
#23569=DIRECTION ( 'NONE',  ( 0.000000000000000000, -0.000000000000000000, -1.000000000000000000 ) ) ;
#23570=CARTESIAN_POINT ( 'NONE',  ( -9.216505592218814158, -7.781333699927420966, -1.500000000000000000 ) ) ;
#23602=CARTESIAN_POINT ( 'NONE',  ( 26.36764545593177544, -31.31467416275353344, -1.500000000000000000 ) ) ;
#23604=EDGE_CURVE ( 'NONE', #18363, #15822, #15941, .T. ) ;
#23628=ORIENTED_EDGE ( 'NONE', *, *, #10956, .F. ) ;
#23633=CARTESIAN_POINT ( 'NONE',  ( -4.163336342344337027E-14, -1.387778780781445676E-14, -1.500000000000000000 ) ) ;
#23641=LINE ( 'NONE', #1682, #22220 ) ;
#23645=EDGE_LOOP ( 'NONE', ( #21090, #8542, #28777, #10757 ) ) ;
#23650=ORIENTED_EDGE ( 'NONE', *, *, #10988, .F. ) ;
#23652=ADVANCED_FACE ( 'NONE', ( #10033 ), #5121, .F. ) ;
#23658=DIRECTION ( 'NONE',  ( -1.000000000000000000, 0.000000000000000000, 0.000000000000000000 ) ) ;
#23684=ORIENTED_EDGE ( 'NONE', *, *, #15271, .T. ) ;
#23686=FACE_OUTER_BOUND ( 'NONE', #21381, .T. ) ;
#23687=LINE ( 'NONE', #12015, #20100 ) ;
#23699=FACE_OUTER_BOUND ( 'NONE', #14377, .T. ) ;
#23708=ORIENTED_EDGE ( 'NONE', *, *, #2724, .T. ) ;
#23721=CARTESIAN_POINT ( 'NONE',  ( 15.57266529552203416, 38.96488032230103471, 1.500000000000000000 ) ) ;
#23725=VERTEX_POINT ( 'NONE', #7388 ) ;
#23729=LINE ( 'NONE', #9862, #30181 ) ;
#23786=EDGE_LOOP ( 'NONE', ( #6540, #12945, #7174, #13686 ) ) ;
#23798=ORIENTED_EDGE ( 'NONE', *, *, #2515, .T. ) ;
#23813=ORIENTED_EDGE ( 'NONE', *, *, #6403, .F. ) ;
#23814=ORIENTED_EDGE ( 'NONE', *, *, #5239, .F. ) ;
#23819=AXIS2_PLACEMENT_3D ( 'NONE', #24680, #29063, #15012 ) ;
#23854=ADVANCED_FACE ( 'NONE', ( #10337 ), #10802, .F. ) ;
#23891=FACE_OUTER_BOUND ( 'NONE', #28829, .T. ) ;
#23895=ADVANCED_FACE ( 'NONE', ( #20318 ), #19849, .F. ) ;
#23896=DIRECTION ( 'NONE',  ( 0.6707505147970024284, -0.7416830501633134842, 0.000000000000000000 ) ) ;
#23906=CARTESIAN_POINT ( 'NONE',  ( -8.860628911697515875, 8.184276679720483116, -1.500000000000000000 ) ) ;
#23927=DIRECTION ( 'NONE',  ( 0.000000000000000000, -0.000000000000000000, -1.000000000000000000 ) ) ;
#23935=ORIENTED_EDGE ( 'NONE', *, *, #29002, .T. ) ;
#23956=DIRECTION ( 'NONE',  ( -0.000000000000000000, -0.000000000000000000, -1.000000000000000000 ) ) ;
#23980=ORIENTED_EDGE ( 'NONE', *, *, #21972, .T. ) ;
#24016=CIRCLE ( 'NONE', #8670, 20.32284676574538906 ) ;
#24018=EDGE_CURVE ( 'NONE', #27621, #6819, #21416, .T. ) ;
#24033=DIRECTION ( 'NONE',  ( -0.000000000000000000, -0.000000000000000000, -1.000000000000000000 ) ) ;
#24037=DIRECTION ( 'NONE',  ( 1.000000000000000000, 0.000000000000000000, 0.000000000000000000 ) ) ;
#24048=VERTEX_POINT ( 'NONE', #7505 ) ;
#24057=ORIENTED_EDGE ( 'NONE', *, *, #15090, .F. ) ;
#24061=ADVANCED_FACE ( 'NONE', ( #23699 ), #12338, .T. ) ;
#24074=ORIENTED_EDGE ( 'NONE', *, *, #25007, .T. ) ;
#24099=AXIS2_PLACEMENT_3D ( 'NONE', #23063, #1428, #3756 ) ;
#24107=CYLINDRICAL_SURFACE ( 'NONE', #28779, 1.447898107987198646 ) ;
#24115=AXIS2_PLACEMENT_3D ( 'NONE', #19307, #28827, #16813 ) ;
#24118=ORIENTED_EDGE ( 'NONE', *, *, #3304, .T. ) ;
#24120=DIRECTION ( 'NONE',  ( 0.6707505147970024284, -0.7416830501633134842, 0.000000000000000000 ) ) ;
#24125=ORIENTED_EDGE ( 'NONE', *, *, #29575, .F. ) ;
#24138=ORIENTED_EDGE ( 'NONE', *, *, #27729, .F. ) ;
#24162=DIRECTION ( 'NONE',  ( 1.000000000000000000, 0.000000000000000000, 0.000000000000000000 ) ) ;
#24163=CARTESIAN_POINT ( 'NONE',  ( -4.163336342344337027E-14, -1.387778780781445676E-14, 1.500000000000000000 ) ) ;
#24170=FACE_OUTER_BOUND ( 'NONE', #30576, .T. ) ;
#24196=CARTESIAN_POINT ( 'NONE',  ( -4.163336342344337027E-14, 1.387778780781445676E-14, 1.500000000000000000 ) ) ;
#24198=CIRCLE ( 'NONE', #17763, 0.7441270634457319844 ) ;
#24206=DIRECTION ( 'NONE',  ( 1.000000000000000000, 0.000000000000000000, 0.000000000000000000 ) ) ;
#24209=ORIENTED_EDGE ( 'NONE', *, *, #8049, .F. ) ;
#24210=EDGE_LOOP ( 'NONE', ( #17500, #29597, #22777, #1856 ) ) ;
#24226=CIRCLE ( 'NONE', #20252, 12.66227964008302287 ) ;
#24227=AXIS2_PLACEMENT_3D ( 'NONE', #514, #10341, #24206 ) ;
#24234=LINE ( 'NONE', #2886, #30536 ) ;
#24258=CARTESIAN_POINT ( 'NONE',  ( -9.301547456646385825, 8.591538895647085283, 1.500000000000000000 ) ) ;
#24265=CIRCLE ( 'NONE', #25273, 1.447898107987170890 ) ;
#24278=EDGE_LOOP ( 'NONE', ( #1719, #5714, #18211, #13712, #29244, #4405 ) ) ;
#24281=CYLINDRICAL_SURFACE ( 'NONE', #27222, 2.061368542273053883 ) ;
#24290=VERTEX_POINT ( 'NONE', #13870 ) ;
#24297=CIRCLE ( 'NONE', #3397, 2.061368542273053883 ) ;
#24302=VERTEX_POINT ( 'NONE', #18696 ) ;
#24331=AXIS2_PLACEMENT_3D ( 'NONE', #9518, #10414, #24746 ) ;
#24339=CARTESIAN_POINT ( 'NONE',  ( -11.21147646446735102, -30.29926891764210595, -1.500000000000000000 ) ) ;
#24346=DIRECTION ( 'NONE',  ( -0.000000000000000000, -0.000000000000000000, -1.000000000000000000 ) ) ;
#24362=DIRECTION ( 'NONE',  ( 0.000000000000000000, -0.000000000000000000, -1.000000000000000000 ) ) ;
#24414=FACE_OUTER_BOUND ( 'NONE', #13024, .T. ) ;
#24436=ORIENTED_EDGE ( 'NONE', *, *, #10703, .T. ) ;
#24441=VERTEX_POINT ( 'NONE', #28677 ) ;
#24462=DIRECTION ( 'NONE',  ( 1.000000000000000000, 0.000000000000000000, 0.000000000000000000 ) ) ;
#24472=ORIENTED_EDGE ( 'NONE', *, *, #25952, .F. ) ;
#24490=FACE_OUTER_BOUND ( 'NONE', #19558, .T. ) ;
#24494=DIRECTION ( 'NONE',  ( -0.000000000000000000, -0.000000000000000000, -1.000000000000000000 ) ) ;
#24500=CARTESIAN_POINT ( 'NONE',  ( -17.84153987719600920, 14.83584055149731284, 1.500000000000000000 ) ) ;
#24507=DIRECTION ( 'NONE',  ( 1.000000000000000000, 2.396195514597832977E-15, 0.000000000000000000 ) ) ;
#24509=CARTESIAN_POINT ( 'NONE',  ( 8.757878075398934925, -7.394122547431893011, 1.500000000000000000 ) ) ;
#24515=ORIENTED_EDGE ( 'NONE', *, *, #25007, .F. ) ;
#24519=CARTESIAN_POINT ( 'NONE',  ( 24.03057240117691862, 26.57182937991349903, 1.500000000000000000 ) ) ;
#24520=VERTEX_POINT ( 'NONE', #5731 ) ;
#24522=VERTEX_POINT ( 'NONE', #29294 ) ;
#24528=PLANE ( 'NONE',  #23819 ) ;
#24537=DIRECTION ( 'NONE',  ( 1.000000000000000000, 0.000000000000000000, 0.000000000000000000 ) ) ;
#24546=CARTESIAN_POINT ( 'NONE',  ( 2.599508007902112006, 14.29059753516471964, -1.500000000000000000 ) ) ;
#24564=FACE_OUTER_BOUND ( 'NONE', #4348, .T. ) ;
#24565=VECTOR ( 'NONE', #13101, 1000.000000000000000 ) ;
#24592=ADVANCED_FACE ( 'NONE', ( #10572 ), #26644, .T. ) ;
#24616=CARTESIAN_POINT ( 'NONE',  ( -25.10445388623454477, 25.60065097860747585, 1.500000000000000000 ) ) ;
#24624=FACE_OUTER_BOUND ( 'NONE', #23556, .T. ) ;
#24628=LINE ( 'NONE', #22748, #27595 ) ;
#24629=DIRECTION ( 'NONE',  ( 1.000000000000000000, 0.000000000000000000, 0.000000000000000000 ) ) ;
#24632=CARTESIAN_POINT ( 'NONE',  ( -4.163336342344337027E-14, -1.387778780781445676E-14, 1.500000000000000000 ) ) ;
#24642=ORIENTED_EDGE ( 'NONE', *, *, #9430, .F. ) ;
#24662=CARTESIAN_POINT ( 'NONE',  ( 24.03057240117691862, 26.57182937991349903, -1.500000000000000000 ) ) ;
#24674=DIRECTION ( 'NONE',  ( -0.7416830501633135952, 0.6707505147970024284, 0.000000000000000000 ) ) ;
#24678=CYLINDRICAL_SURFACE ( 'NONE', #18428, 28.20443790117963800 ) ;
#24680=CARTESIAN_POINT ( 'NONE',  ( 1.073881485057738949, 0.9711784013061123266, 1.500000000000000000 ) ) ;
#24685=AXIS2_PLACEMENT_3D ( 'NONE', #25480, #4101, #24462 ) ;
#24687=CARTESIAN_POINT ( 'NONE',  ( 2.599508007902112006, -14.29059753516471964, -1.500000000000000000 ) ) ;
#24711=ORIENTED_EDGE ( 'NONE', *, *, #28807, .T. ) ;
#24716=DIRECTION ( 'NONE',  ( -0.000000000000000000, 0.000000000000000000, 1.000000000000000000 ) ) ;
#24722=DIRECTION ( 'NONE',  ( -0.000000000000000000, -0.000000000000000000, -1.000000000000000000 ) ) ;
#24746=DIRECTION ( 'NONE',  ( 1.000000000000000000, 0.000000000000000000, 0.000000000000000000 ) ) ;
#24770=FACE_BOUND ( 'NONE', #29983, .T. ) ;
#24781=VERTEX_POINT ( 'NONE', #8665 ) ;
#24795=EDGE_CURVE ( 'NONE', #19078, #28942, #22461, .T. ) ;
#24796=CARTESIAN_POINT ( 'NONE',  ( 1.073881485057738949, 0.9711784013061123266, -1.500000000000000000 ) ) ;
#24804=AXIS2_PLACEMENT_3D ( 'NONE', #29108, #4941, #18989 ) ;
#24809=PLANE ( 'NONE',  #21529 ) ;
#24824=DIRECTION ( 'NONE',  ( -0.000000000000000000, 0.000000000000000000, 1.000000000000000000 ) ) ;
#24825=VERTEX_POINT ( 'NONE', #29311 ) ;
#24833=CARTESIAN_POINT ( 'NONE',  ( 0.000000000000000000, 0.000000000000000000, 1.500000000000000000 ) ) ;
#24844=EDGE_CURVE ( 'NONE', #27621, #24302, #16984, .T. ) ;
#24881=DIRECTION ( 'NONE',  ( 1.000000000000000000, 0.000000000000000000, 0.000000000000000000 ) ) ;
#24884=AXIS2_PLACEMENT_3D ( 'NONE', #4223, #15776, #18729 ) ;
#24885=CARTESIAN_POINT ( 'NONE',  ( 8.419710366748642372, 7.777014463793876509, -1.500000000000000000 ) ) ;
#24888=CARTESIAN_POINT ( 'NONE',  ( -4.163336342344337027E-14, 1.387778780781445676E-14, -1.500000000000000000 ) ) ;
#24890=EDGE_CURVE ( 'NONE', #16799, #3576, #26826, .T. ) ;
#24897=DIRECTION ( 'NONE',  ( 1.000000000000000000, 0.000000000000000000, 0.000000000000000000 ) ) ;
#24904=CYLINDRICAL_SURFACE ( 'NONE', #4120, 2.061368542273053883 ) ;
#24905=ORIENTED_EDGE ( 'NONE', *, *, #9045, .F. ) ;
#24914=VERTEX_POINT ( 'NONE', #24616 ) ;
#24929=DIRECTION ( 'NONE',  ( 0.000000000000000000, -0.000000000000000000, -1.000000000000000000 ) ) ;
#24933=FACE_BOUND ( 'NONE', #24278, .T. ) ;
#24947=FACE_OUTER_BOUND ( 'NONE', #13118, .T. ) ;
#24959=EDGE_LOOP ( 'NONE', ( #7286, #22417, #1277, #26029, #1462, #6201, #13718, #17681, #15352, #21566, #15512, #18161, #15919, #4329, #28487, #21927, #29052, #2668, #23813, #25721, #29131, #4147, #23798, #22217, #6387, #28022 ) ) ;
#24978=DIRECTION ( 'NONE',  ( 1.000000000000000000, 0.000000000000000000, 0.000000000000000000 ) ) ;
#24990=ORIENTED_EDGE ( 'NONE', *, *, #192, .F. ) ;
#24992=CARTESIAN_POINT ( 'NONE',  ( -4.163336342344337027E-14, -1.387778780781445676E-14, 1.500000000000000000 ) ) ;
#24995=CARTESIAN_POINT ( 'NONE',  ( 3.637110358602580362, -19.99473753024311762, 1.500000000000000000 ) ) ;
#25000=DIRECTION ( 'NONE',  ( -0.000000000000000000, -0.000000000000000000, -1.000000000000000000 ) ) ;
#25007=EDGE_CURVE ( 'NONE', #21157, #7845, #8870, .T. ) ;
#25009=EDGE_CURVE ( 'NONE', #30777, #4361, #30226, .T. ) ;
#25028=EDGE_CURVE ( 'NONE', #25685, #22720, #27261, .T. ) ;
#25032=ORIENTED_EDGE ( 'NONE', *, *, #7675, .T. ) ;
#25037=ORIENTED_EDGE ( 'NONE', *, *, #4625, .T. ) ;
#25052=ORIENTED_EDGE ( 'NONE', *, *, #30696, .T. ) ;
#25070=ORIENTED_EDGE ( 'NONE', *, *, #12082, .F. ) ;
#25087=CARTESIAN_POINT ( 'NONE',  ( -3.515970705488605130, 17.06554576617236307, 1.500000000000000000 ) ) ;
#25089=AXIS2_PLACEMENT_3D ( 'NONE', #1123, #8474, #15616 ) ;
#25096=CARTESIAN_POINT ( 'NONE',  ( 17.26937953831880534, -14.36006998371588317, 1.500000000000000000 ) ) ;
#25105=DIRECTION ( 'NONE',  ( -0.000000000000000000, -0.000000000000000000, -1.000000000000000000 ) ) ;
#25128=ORIENTED_EDGE ( 'NONE', *, *, #19324, .F. ) ;
#25145=VERTEX_POINT ( 'NONE', #10233 ) ;
#25146=CARTESIAN_POINT ( 'NONE',  ( 17.84153987719590972, -14.83584055149750114, 1.500000000000000000 ) ) ;
#25149=DIRECTION ( 'NONE',  ( -1.000000000000000000, 0.000000000000000000, 0.000000000000000000 ) ) ;
#25152=LINE ( 'NONE', #18148, #9118 ) ;
#25158=DIRECTION ( 'NONE',  ( 1.000000000000000000, 0.000000000000000000, 0.000000000000000000 ) ) ;
#25181=DIRECTION ( 'NONE',  ( -0.7416830501633041584, 0.6707505147970128645, 0.000000000000000000 ) ) ;
#25189=CARTESIAN_POINT ( 'NONE',  ( -26.36764545593177544, 31.31467416275353344, 1.500000000000000000 ) ) ;
#25198=DIRECTION ( 'NONE',  ( -0.000000000000000000, -0.000000000000000000, -1.000000000000000000 ) ) ;
#25201=CIRCLE ( 'NONE', #20696, 11.46182693247429718 ) ;
#25234=DIRECTION ( 'NONE',  ( -0.000000000000000000, -0.000000000000000000, -1.000000000000000000 ) ) ;
#25245=EDGE_CURVE ( 'NONE', #3989, #3010, #20205, .T. ) ;
#25264=ORIENTED_EDGE ( 'NONE', *, *, #26374, .F. ) ;
#25273=AXIS2_PLACEMENT_3D ( 'NONE', #10980, #6739, #20626 ) ;
#25274=ORIENTED_EDGE ( 'NONE', *, *, #10561, .F. ) ;
#25275=CIRCLE ( 'NONE', #871, 0.6002263538043630664 ) ;
#25290=FACE_OUTER_BOUND ( 'NONE', #26265, .T. ) ;
#25342=AXIS2_PLACEMENT_3D ( 'NONE', #15304, #6105, #1284 ) ;
#25349=CIRCLE ( 'NONE', #2441, 0.7441270634457337607 ) ;
#25356=EDGE_CURVE ( 'NONE', #21157, #27347, #27553, .T. ) ;
#25357=DIRECTION ( 'NONE',  ( -0.000000000000000000, -0.000000000000000000, -1.000000000000000000 ) ) ;
#25373=CARTESIAN_POINT ( 'NONE',  ( -3.515970705488605130, -17.06554576617236307, -1.500000000000000000 ) ) ;
#25383=AXIS2_PLACEMENT_3D ( 'NONE', #29847, #10494, #20005 ) ;
#25401=EDGE_CURVE ( 'NONE', #16767, #27365, #23317, .T. ) ;
#25408=DIRECTION ( 'NONE',  ( -0.000000000000000000, 0.000000000000000000, 1.000000000000000000 ) ) ;
#25411=ORIENTED_EDGE ( 'NONE', *, *, #10385, .F. ) ;
#25418=LINE ( 'NONE', #1854, #15661 ) ;
#25426=EDGE_CURVE ( 'NONE', #15589, #1105, #7560, .T. ) ;
#25434=EDGE_CURVE ( 'NONE', #16733, #30322, #30634, .T. ) ;
#25443=CARTESIAN_POINT ( 'NONE',  ( 24.03057240117691862, 26.57182937991349903, 1.500000000000000000 ) ) ;
#25471=DIRECTION ( 'NONE',  ( -0.000000000000000000, -0.000000000000000000, -1.000000000000000000 ) ) ;
#25480=CARTESIAN_POINT ( 'NONE',  ( -4.163336342344337027E-14, -1.387778780781445676E-14, -1.500000000000000000 ) ) ;
#25481=FACE_OUTER_BOUND ( 'NONE', #27239, .T. ) ;
#25490=VERTEX_POINT ( 'NONE', #25970 ) ;
#25505=ORIENTED_EDGE ( 'NONE', *, *, #25401, .F. ) ;
#25515=FACE_OUTER_BOUND ( 'NONE', #22245, .T. ) ;
#25517=DIRECTION ( 'NONE',  ( -0.000000000000000000, 0.000000000000000000, 1.000000000000000000 ) ) ;
#25528=ORIENTED_EDGE ( 'NONE', *, *, #10538, .T. ) ;
#25557=EDGE_CURVE ( 'NONE', #8512, #20433, #23103, .T. ) ;
#25568=ORIENTED_EDGE ( 'NONE', *, *, #8197, .F. ) ;
#25583=CIRCLE ( 'NONE', #26063, 2.898871837527149609 ) ;
#25585=DIRECTION ( 'NONE',  ( 0.000000000000000000, -0.000000000000000000, -1.000000000000000000 ) ) ;
#25587=DIRECTION ( 'NONE',  ( 1.000000000000000000, 0.000000000000000000, 0.000000000000000000 ) ) ;
#25607=VECTOR ( 'NONE', #21907, 1000.000000000000000 ) ;
#25616=ORIENTED_EDGE ( 'NONE', *, *, #2110, .T. ) ;
#25634=CARTESIAN_POINT ( 'NONE',  ( -26.36764545593177544, -31.31467416275353344, -1.500000000000000000 ) ) ;
#25639=LINE ( 'NONE', #13930, #23532 ) ;
#25652=ORIENTED_EDGE ( 'NONE', *, *, #29014, .F. ) ;
#25656=CARTESIAN_POINT ( 'NONE',  ( -3.221450758838616757, 1.621276839356792454, 1.500000000000000000 ) ) ;
#25666=AXIS2_PLACEMENT_3D ( 'NONE', #5193, #14856, #29671 ) ;
#25668=DIRECTION ( 'NONE',  ( 0.000000000000000000, -0.000000000000000000, -1.000000000000000000 ) ) ;
#25675=DIRECTION ( 'NONE',  ( -0.000000000000000000, -0.000000000000000000, -1.000000000000000000 ) ) ;
#25685=VERTEX_POINT ( 'NONE', #7037 ) ;
#25687=AXIS2_PLACEMENT_3D ( 'NONE', #24662, #5494, #24507 ) ;
#25698=CARTESIAN_POINT ( 'NONE',  ( 14.83584055149749759, 17.84153987719500734, 1.500000000000000000 ) ) ;
#25705=VERTEX_POINT ( 'NONE', #14824 ) ;
#25714=AXIS2_PLACEMENT_3D ( 'NONE', #11199, #30383, #18992 ) ;
#25717=CARTESIAN_POINT ( 'NONE',  ( 11.21147646446735102, 30.29926891764210595, 1.500000000000000000 ) ) ;
#25721=ORIENTED_EDGE ( 'NONE', *, *, #21194, .F. ) ;
#25724=AXIS2_PLACEMENT_3D ( 'NONE', #26387, #24494, #14979 ) ;
#25733=ADVANCED_FACE ( 'NONE', ( #24170 ), #5008, .F. ) ;
#25738=VERTEX_POINT ( 'NONE', #24339 ) ;
#25739=ORIENTED_EDGE ( 'NONE', *, *, #14502, .T. ) ;
#25772=DIRECTION ( 'NONE',  ( -0.000000000000000000, 0.000000000000000000, 1.000000000000000000 ) ) ;
#25782=CARTESIAN_POINT ( 'NONE',  ( -3.515970705488605130, 17.06554576617236307, -1.500000000000000000 ) ) ;
#25787=AXIS2_PLACEMENT_3D ( 'NONE', #6449, #25772, #30447 ) ;
#25804=ORIENTED_EDGE ( 'NONE', *, *, #4774, .F. ) ;
#25815=LINE ( 'NONE', #13957, #5279 ) ;
#25868=ORIENTED_EDGE ( 'NONE', *, *, #10687, .F. ) ;
#25879=CYLINDRICAL_SURFACE ( 'NONE', #3475, 37.60050224823048381 ) ;
#25882=ORIENTED_EDGE ( 'NONE', *, *, #19668, .F. ) ;
#25889=ORIENTED_EDGE ( 'NONE', *, *, #953, .T. ) ;
#25894=ORIENTED_EDGE ( 'NONE', *, *, #15887, .T. ) ;
#25905=CYLINDRICAL_SURFACE ( 'NONE', #30633, 0.6002263538043648428 ) ;
#25910=ORIENTED_EDGE ( 'NONE', *, *, #3100, .T. ) ;
#25922=CARTESIAN_POINT ( 'NONE',  ( -28.34828976096172681, 29.18752572968383419, 1.500000000000000000 ) ) ;
#25937=EDGE_CURVE ( 'NONE', #23361, #5698, #20544, .T. ) ;
#25952=EDGE_CURVE ( 'NONE', #3349, #27621, #20849, .T. ) ;
#25965=CARTESIAN_POINT ( 'NONE',  ( 23.17581250239727808, -34.50630206824671831, -1.499999999999999778 ) ) ;
#25970=CARTESIAN_POINT ( 'NONE',  ( -8.757878075398936701, -7.394122547431892123, 1.500000000000000000 ) ) ;
#25981=EDGE_CURVE ( 'NONE', #7027, #29776, #252, .T. ) ;
#26012=ORIENTED_EDGE ( 'NONE', *, *, #17781, .T. ) ;
#26021=CYLINDRICAL_SURFACE ( 'NONE', #16669, 11.46182693247429718 ) ;
#26022=VERTEX_POINT ( 'NONE', #26460 ) ;
#26029=ORIENTED_EDGE ( 'NONE', *, *, #3160, .F. ) ;
#26033=CARTESIAN_POINT ( 'NONE',  ( -8.860628911697515875, 8.184276679720483116, 1.500000000000000000 ) ) ;
#26038=CARTESIAN_POINT ( 'NONE',  ( -43.34097750826428097, 11.89502811014148342, 1.500000000000000444 ) ) ;
#26041=LINE ( 'NONE', #16217, #15238 ) ;
#26043=CARTESIAN_POINT ( 'NONE',  ( -26.83043119477639493, -8.695877139419037505, 1.500000000000000000 ) ) ;
#26046=EDGE_CURVE ( 'NONE', #30031, #21650, #2447, .T. ) ;
#26051=CARTESIAN_POINT ( 'NONE',  ( -28.34828976096172681, -29.18752572968383419, 1.500000000000000000 ) ) ;
#26063=AXIS2_PLACEMENT_3D ( 'NONE', #8924, #9517, #11866 ) ;
#26077=ORIENTED_EDGE ( 'NONE', *, *, #22939, .F. ) ;
#26085=ORIENTED_EDGE ( 'NONE', *, *, #6552, .T. ) ;
#26092=ORIENTED_EDGE ( 'NONE', *, *, #15271, .F. ) ;
#26094=CARTESIAN_POINT ( 'NONE',  ( -28.34828976096172681, -29.18752572968383063, -1.500000000000000000 ) ) ;
#26117=EDGE_CURVE ( 'NONE', #6039, #30777, #2755, .T. ) ;
#26126=ORIENTED_EDGE ( 'NONE', *, *, #25981, .T. ) ;
#26143=VECTOR ( 'NONE', #12254, 1000.000000000000000 ) ;
#26149=EDGE_CURVE ( 'NONE', #26677, #15822, #1185, .T. ) ;
#26151=ADVANCED_FACE ( 'NONE', ( #7904 ), #19906, .F. ) ;
#26156=ORIENTED_EDGE ( 'NONE', *, *, #6915, .F. ) ;
#26175=CARTESIAN_POINT ( 'NONE',  ( 0.000000000000000000, 0.000000000000000000, 1.500000000000000000 ) ) ;
#26183=CARTESIAN_POINT ( 'NONE',  ( 24.03057240117691862, -26.57182937991349903, -1.500000000000000000 ) ) ;
#26194=EDGE_LOOP ( 'NONE', ( #29705, #8013, #27267, #3437 ) ) ;
#26212=ADVANCED_FACE ( 'NONE', ( #15670 ), #1945, .F. ) ;
#26219=CARTESIAN_POINT ( 'NONE',  ( -24.03057240117691862, -26.57182937991349903, 1.500000000000000000 ) ) ;
#26241=EDGE_LOOP ( 'NONE', ( #12451, #29418, #20496, #19520 ) ) ;
#26265=EDGE_LOOP ( 'NONE', ( #8404, #20128, #7869, #29399 ) ) ;
#26270=CARTESIAN_POINT ( 'NONE',  ( 3.221450758838616757, 1.621276839356792454, 1.500000000000000000 ) ) ;
#26272=AXIS2_PLACEMENT_3D ( 'NONE', #955, #10465, #19655 ) ;
#26282=FACE_OUTER_BOUND ( 'NONE', #30409, .T. ) ;
#26304=VECTOR ( 'NONE', #18488, 1000.000000000000000 ) ;
#26305=CYLINDRICAL_SURFACE ( 'NONE', #30723, 0.7441270634456955690 ) ;
#26311=CARTESIAN_POINT ( 'NONE',  ( -4.163336342344337027E-14, -1.387778780781445676E-14, 1.500000000000000000 ) ) ;
#26313=DIRECTION ( 'NONE',  ( -1.000000000000000000, 0.000000000000000000, 0.000000000000000000 ) ) ;
#26320=EDGE_LOOP ( 'NONE', ( #1514, #22344, #17958, #9173 ) ) ;
#26324=ORIENTED_EDGE ( 'NONE', *, *, #9991, .F. ) ;
#26353=CARTESIAN_POINT ( 'NONE',  ( -28.34828976096172681, 29.18752572968383419, 1.500000000000000000 ) ) ;
#26355=CIRCLE ( 'NONE', #11917, 12.66227964008302287 ) ;
#26374=EDGE_CURVE ( 'NONE', #9927, #27254, #9577, .T. ) ;
#26376=VERTEX_POINT ( 'NONE', #12699 ) ;
#26381=EDGE_CURVE ( 'NONE', #30322, #18363, #20530, .T. ) ;
#26387=CARTESIAN_POINT ( 'NONE',  ( -4.163336342344337027E-14, 1.387778780781445676E-14, 1.500000000000000000 ) ) ;
#26391=CARTESIAN_POINT ( 'NONE',  ( -26.36764545593178255, -31.31467416275353344, 1.500000000000000000 ) ) ;
#26460=CARTESIAN_POINT ( 'NONE',  ( 26.31795596221988376, 10.51822134874671022, -1.500000000000000000 ) ) ;
#26476=CARTESIAN_POINT ( 'NONE',  ( -26.44644203219470668, 9.801837641955994940, 1.500000000000000000 ) ) ;
#26486=DIRECTION ( 'NONE',  ( 0.6707505147970089787, -0.7416830501633076000, 0.000000000000000000 ) ) ;
#26492=ORIENTED_EDGE ( 'NONE', *, *, #15630, .F. ) ;
#26498=CARTESIAN_POINT ( 'NONE',  ( -26.83043119477639493, -8.695877139419037505, -1.500000000000000000 ) ) ;
#26511=ADVANCED_FACE ( 'NONE', ( #13763 ), #8632, .T. ) ;
#26518=EDGE_CURVE ( 'NONE', #6039, #10630, #3639, .T. ) ;
#26521=CYLINDRICAL_SURFACE ( 'NONE', #6759, 20.32284676574536064 ) ;
#26526=ADVANCED_FACE ( 'NONE', ( #17841 ), #15481, .T. ) ;
#26533=CIRCLE ( 'NONE', #3628, 23.20393738267273420 ) ;
#26537=DIRECTION ( 'NONE',  ( 0.7416830501633076000, -0.6707505147970089787, 0.000000000000000000 ) ) ;
#26544=ORIENTED_EDGE ( 'NONE', *, *, #429, .F. ) ;
#26547=EDGE_CURVE ( 'NONE', #15589, #9342, #23415, .T. ) ;
#26551=ORIENTED_EDGE ( 'NONE', *, *, #4046, .F. ) ;
#26564=CIRCLE ( 'NONE', #3140, 21.71568325578132530 ) ;
#26568=CYLINDRICAL_SURFACE ( 'NONE', #25666, 0.7441270634457163302 ) ;
#26591=ORIENTED_EDGE ( 'NONE', *, *, #26149, .F. ) ;
#26604=CARTESIAN_POINT ( 'NONE',  ( 30.31220697679117038, 11.23460505553742550, 1.500000000000000000 ) ) ;
#26610=ORIENTED_EDGE ( 'NONE', *, *, #23049, .T. ) ;
#26623=FACE_OUTER_BOUND ( 'NONE', #26320, .T. ) ;
#26635=ORIENTED_EDGE ( 'NONE', *, *, #9738, .T. ) ;
#26644=CYLINDRICAL_SURFACE ( 'NONE', #25, 28.20443790117963800 ) ;
#26647=EDGE_LOOP ( 'NONE', ( #19758, #12484, #3229, #14224, #28167 ) ) ;
#26653=AXIS2_PLACEMENT_3D ( 'NONE', #9709, #28747, #14398 ) ;
#26657=DIRECTION ( 'NONE',  ( -0.000000000000000000, 0.000000000000000000, 1.000000000000000000 ) ) ;
#26664=AXIS2_PLACEMENT_3D ( 'NONE', #5304, #156, #24162 ) ;
#26671=VERTEX_POINT ( 'NONE', #4699 ) ;
#26677=VERTEX_POINT ( 'NONE', #14054 ) ;
#26680=FACE_OUTER_BOUND ( 'NONE', #7570, .T. ) ;
#26695=DIRECTION ( 'NONE',  ( -0.000000000000000000, -0.000000000000000000, -1.000000000000000000 ) ) ;
#26698=DIRECTION ( 'NONE',  ( 1.000000000000000000, 0.000000000000000000, 0.000000000000000000 ) ) ;
#26703=LINE ( 'NONE', #5333, #22206 ) ;
#26715=FACE_OUTER_BOUND ( 'NONE', #21715, .T. ) ;
#26717=ORIENTED_EDGE ( 'NONE', *, *, #21167, .T. ) ;
#26720=EDGE_CURVE ( 'NONE', #9920, #19640, #13100, .T. ) ;
#26731=ORIENTED_EDGE ( 'NONE', *, *, #10536, .T. ) ;
#26735=CARTESIAN_POINT ( 'NONE',  ( 15.57266529552203416, -38.96488032230103471, 1.500000000000000000 ) ) ;
#26739=ORIENTED_EDGE ( 'NONE', *, *, #11751, .T. ) ;
#26768=AXIS2_PLACEMENT_3D ( 'NONE', #7336, #16846, #7492 ) ;
#26769=CARTESIAN_POINT ( 'NONE',  ( 1.073881485057738949, -0.9711784013061123266, -1.500000000000000000 ) ) ;
#26770=ADVANCED_FACE ( 'NONE', ( #2826 ), #24809, .F. ) ;
#26824=FACE_OUTER_BOUND ( 'NONE', #15892, .T. ) ;
#26826=LINE ( 'NONE', #14793, #3554 ) ;
#26834=DIRECTION ( 'NONE',  ( 1.000000000000000000, 0.000000000000000000, 0.000000000000000000 ) ) ;
#26852=CARTESIAN_POINT ( 'NONE',  ( 1.073881485057738949, -0.9711784013061123266, 1.500000000000000000 ) ) ;
#26853=VECTOR ( 'NONE', #25675, 1000.000000000000000 ) ;
#26872=DIRECTION ( 'NONE',  ( -0.000000000000000000, -0.000000000000000000, -1.000000000000000000 ) ) ;
#26884=ORIENTED_EDGE ( 'NONE', *, *, #3465, .F. ) ;
#26890=CYLINDRICAL_SURFACE ( 'NONE', #18373, 1.447898107987198646 ) ;
#26896=ORIENTED_EDGE ( 'NONE', *, *, #7675, .F. ) ;
#26907=ADVANCED_FACE ( 'NONE', ( #11081 ), #6553, .F. ) ;
#26918=PRODUCT_CONTEXT ( 'NONE', #5195, 'mechanical' ) ;
#26926=EDGE_CURVE ( 'NONE', #23449, #27382, #1265, .T. ) ;
#26935=APPLICATION_CONTEXT ( 'automotive_design' ) ;
#26949=CARTESIAN_POINT ( 'NONE',  ( 3.637110358602580362, -19.99473753024311762, 1.500000000000000000 ) ) ;
#26950=VERTEX_POINT ( 'NONE', #15442 ) ;
#26953=DIRECTION ( 'NONE',  ( 1.000000000000000000, 0.000000000000000000, 0.000000000000000000 ) ) ;
#26955=EDGE_CURVE ( 'NONE', #27927, #24825, #10773, .T. ) ;
#26962=AXIS2_PLACEMENT_3D ( 'NONE', #10349, #19860, #10501 ) ;
#26969=CARTESIAN_POINT ( 'NONE',  ( 43.34097750826426676, -11.89502811014149941, 1.500000000000000000 ) ) ;
#26988=VERTEX_POINT ( 'NONE', #22926 ) ;
#26994=DIRECTION ( 'NONE',  ( -0.000000000000000000, -0.000000000000000000, -1.000000000000000000 ) ) ;
#27002=CARTESIAN_POINT ( 'NONE',  ( 26.36764545593179676, 31.31467416275351923, 1.500000000000000000 ) ) ;
#27039=ORIENTED_EDGE ( 'NONE', *, *, #14502, .F. ) ;
#27040=CARTESIAN_POINT ( 'NONE',  ( 17.26937953831880534, -14.36006998371588317, -1.500000000000000000 ) ) ;
#27058=ORIENTED_EDGE ( 'NONE', *, *, #13187, .F. ) ;
#27074=DIRECTION ( 'NONE',  ( -0.000000000000000000, 0.000000000000000000, 1.000000000000000000 ) ) ;
#27093=ORIENTED_EDGE ( 'NONE', *, *, #20469, .F. ) ;
#27118=EDGE_CURVE ( 'NONE', #22347, #7027, #9499, .T. ) ;
#27127=ORIENTED_EDGE ( 'NONE', *, *, #26720, .T. ) ;
#27131=CYLINDRICAL_SURFACE ( 'NONE', #6118, 0.6002263538043630664 ) ;
#27154=DIRECTION ( 'NONE',  ( 1.000000000000000000, 0.000000000000000000, 0.000000000000000000 ) ) ;
#27190=DIRECTION ( 'NONE',  ( 1.000000000000000000, 0.000000000000000000, 0.000000000000000000 ) ) ;
#27192=DIRECTION ( 'NONE',  ( 1.000000000000000000, 0.000000000000000000, 0.000000000000000000 ) ) ;
#27216=ORIENTED_EDGE ( 'NONE', *, *, #6930, .F. ) ;
#27221=CYLINDRICAL_SURFACE ( 'NONE', #9357, 23.20393738267342698 ) ;
#27222=AXIS2_PLACEMENT_3D ( 'NONE', #2929, #12447, #28966 ) ;
#27223=CIRCLE ( 'NONE', #14768, 20.32284676574538906 ) ;
#27229=CARTESIAN_POINT ( 'NONE',  ( -4.100931858250869588, 19.90478481566557178, 1.500000000000000000 ) ) ;
#27232=CYLINDRICAL_SURFACE ( 'NONE', #317, 23.20393738267338790 ) ;
#27234=CARTESIAN_POINT ( 'NONE',  ( -28.34828976096172681, -29.18752572968383419, -1.500000000000000000 ) ) ;
#27239=EDGE_LOOP ( 'NONE', ( #19159, #17849, #5049, #17928 ) ) ;
#27252=LINE ( 'NONE', #13071, #2436 ) ;
#27254=VERTEX_POINT ( 'NONE', #5597 ) ;
#27259=CIRCLE ( 'NONE', #29750, 23.20393738267342698 ) ;
#27261=( BOUNDED_CURVE ( )  B_SPLINE_CURVE ( 3, ( #30522, #28655, #28504, #16797 ),
 .UNSPECIFIED., .F., .T. ) 
 B_SPLINE_CURVE_WITH_KNOTS ( ( 4, 4 ),
 ( 3.955359442064654285, 5.469418518704724619 ),
 .UNSPECIFIED. ) 
 CURVE ( )  GEOMETRIC_REPRESENTATION_ITEM ( )  RATIONAL_B_SPLINE_CURVE ( ( 1.000000000000000000, 0.8179194830933629312, 0.8179194830933629312, 1.000000000000000000 ) ) 
 REPRESENTATION_ITEM ( '' )  );
#27267=ORIENTED_EDGE ( 'NONE', *, *, #1264, .F. ) ;
#27273=VECTOR ( 'NONE', #15936, 1000.000000000000000 ) ;
#27291=VERTEX_POINT ( 'NONE', #19943 ) ;
#27345=VECTOR ( 'NONE', #7252, 1000.000000000000114 ) ;
#27347=VERTEX_POINT ( 'NONE', #1537 ) ;
#27352=VERTEX_POINT ( 'NONE', #28181 ) ;
#27353=DIRECTION ( 'NONE',  ( -0.000000000000000000, -0.000000000000000000, -1.000000000000000000 ) ) ;
#27362=CARTESIAN_POINT ( 'NONE',  ( 23.17581250239727808, -34.50630206824672541, 1.499999999999999778 ) ) ;
#27365=VERTEX_POINT ( 'NONE', #20854 ) ;
#27374=AXIS2_PLACEMENT_3D ( 'NONE', #28743, #24362, #14689 ) ;
#27382=VERTEX_POINT ( 'NONE', #16339 ) ;
#27391=FACE_OUTER_BOUND ( 'NONE', #12014, .T. ) ;
#27393=AXIS2_PLACEMENT_3D ( 'NONE', #23410, #23553, #11717 ) ;
#27416=ORIENTED_EDGE ( 'NONE', *, *, #4625, .F. ) ;
#27427=ORIENTED_EDGE ( 'NONE', *, *, #3304, .F. ) ;
#27429=VERTEX_POINT ( 'NONE', #9160 ) ;
#27445=VERTEX_POINT ( 'NONE', #18674 ) ;
#27469=EDGE_CURVE ( 'NONE', #9122, #15261, #28033, .T. ) ;
#27472=ORIENTED_EDGE ( 'NONE', *, *, #652, .F. ) ;
#27481=CARTESIAN_POINT ( 'NONE',  ( 14.83584055149749759, 17.84153987719500734, 1.500000000000000000 ) ) ;
#27483=AXIS2_PLACEMENT_3D ( 'NONE', #15001, #12527, #17351 ) ;
#27489=EDGE_CURVE ( 'NONE', #8808, #27445, #18388, .T. ) ;
#27492=VECTOR ( 'NONE', #5872, 1000.000000000000000 ) ;
#27493=DIRECTION ( 'NONE',  ( -0.000000000000000000, -0.000000000000000000, -1.000000000000000000 ) ) ;
#27498=VERTEX_POINT ( 'NONE', #26735 ) ;
#27510=CARTESIAN_POINT ( 'NONE',  ( 11.21147646446735102, 30.29926891764210595, 1.500000000000000000 ) ) ;
#27525=DIRECTION ( 'NONE',  ( 1.000000000000000000, 0.000000000000000000, 0.000000000000000000 ) ) ;
#27534=EDGE_CURVE ( 'NONE', #27498, #3343, #8320, .T. ) ;
#27537=DIRECTION ( 'NONE',  ( -0.000000000000000000, -0.000000000000000000, -1.000000000000000000 ) ) ;
#27539=ORIENTED_EDGE ( 'NONE', *, *, #15090, .T. ) ;
#27542=CARTESIAN_POINT ( 'NONE',  ( -17.79239818699324616, -14.89473990422481187, 1.500000000000000000 ) ) ;
#27550=DIRECTION ( 'NONE',  ( 0.000000000000000000, -0.000000000000000000, -1.000000000000000000 ) ) ;
#27553=LINE ( 'NONE', #6179, #4062 ) ;
#27566=VECTOR ( 'NONE', #23349, 1000.000000000000000 ) ;
#27569=ORIENTED_EDGE ( 'NONE', *, *, #21582, .F. ) ;
#27595=VECTOR ( 'NONE', #15256, 1000.000000000000000 ) ;
#27604=CARTESIAN_POINT ( 'NONE',  ( -26.36764545593177544, -31.31467416275353344, 1.500000000000000000 ) ) ;
#27612=ORIENTED_EDGE ( 'NONE', *, *, #7849, .T. ) ;
#27621=VERTEX_POINT ( 'NONE', #24687 ) ;
#27625=ORIENTED_EDGE ( 'NONE', *, *, #7435, .T. ) ;
#27637=CARTESIAN_POINT ( 'NONE',  ( 26.44644203219471379, 9.801837641955973623, 1.500000000000000000 ) ) ;
#27655=FACE_OUTER_BOUND ( 'NONE', #8731, .T. ) ;
#27667=ORIENTED_EDGE ( 'NONE', *, *, #27924, .T. ) ;
#27685=EDGE_CURVE ( 'NONE', #10191, #3847, #25152, .T. ) ;
#27688=CARTESIAN_POINT ( 'NONE',  ( -14.83584055149731817, -17.84153987719691514, 1.500000000000000000 ) ) ;
#27694=ADVANCED_FACE ( 'NONE', ( #29999 ), #16108, .T. ) ;
#27707=ORIENTED_EDGE ( 'NONE', *, *, #3226, .F. ) ;
#27710=EDGE_CURVE ( 'NONE', #21029, #19394, #11435, .T. ) ;
#27712=EDGE_CURVE ( 'NONE', #24914, #6039, #5341, .T. ) ;
#27729=EDGE_CURVE ( 'NONE', #24441, #20436, #24265, .T. ) ;
#27732=AXIS2_PLACEMENT_3D ( 'NONE', #14457, #19444, #21624 ) ;
#27736=CYLINDRICAL_SURFACE ( 'NONE', #6745, 28.20443790117971261 ) ;
#27740=CARTESIAN_POINT ( 'NONE',  ( -17.84153987719600920, 14.83584055149731284, 1.500000000000000000 ) ) ;
#27746=VECTOR ( 'NONE', #13516, 1000.000000000000000 ) ;
#27803=VECTOR ( 'NONE', #16642, 1000.000000000000000 ) ;
#27807=ORIENTED_EDGE ( 'NONE', *, *, #27489, .F. ) ;
#27813=EDGE_LOOP ( 'NONE', ( #19553, #1876, #23935, #6585 ) ) ;
#27823=ORIENTED_EDGE ( 'NONE', *, *, #23249, .F. ) ;
#27824=AXIS2_PLACEMENT_3D ( 'NONE', #23451, #13956, #1951 ) ;
#27825=AXIS2_PLACEMENT_3D ( 'NONE', #12005, #4818, #30703 ) ;
#27833=ORIENTED_EDGE ( 'NONE', *, *, #6552, .F. ) ;
#27846=CIRCLE ( 'NONE', #24331, 2.061368542273053883 ) ;
#27847=DIRECTION ( 'NONE',  ( 1.000000000000000000, 0.000000000000000000, 0.000000000000000000 ) ) ;
#27851=CARTESIAN_POINT ( 'NONE',  ( -14.36006998371493637, -17.26937953831884442, -1.500000000000000000 ) ) ;
#27852=VECTOR ( 'NONE', #10298, 1000.000000000000000 ) ;
#27862=DIRECTION ( 'NONE',  ( -0.000000000000000000, -0.000000000000000000, -1.000000000000000000 ) ) ;
#27886=ORIENTED_EDGE ( 'NONE', *, *, #12257, .T. ) ;
#27893=EDGE_CURVE ( 'NONE', #9405, #9920, #6893, .T. ) ;
#27895=EDGE_CURVE ( 'NONE', #4581, #16359, #17297, .T. ) ;
#27924=EDGE_CURVE ( 'NONE', #20068, #3010, #13329, .T. ) ;
#27925=ORIENTED_EDGE ( 'NONE', *, *, #16409, .T. ) ;
#27926=AXIS2_PLACEMENT_3D ( 'NONE', #29873, #6298, #27525 ) ;
#27927=VERTEX_POINT ( 'NONE', #25922 ) ;
#27956=VERTEX_POINT ( 'NONE', #4551 ) ;
#27968=CYLINDRICAL_SURFACE ( 'NONE', #10158, 2.898871837527149165 ) ;
#27972=CARTESIAN_POINT ( 'NONE',  ( 14.41708049311143469, -17.22181377297010130, -1.500000000000000000 ) ) ;
#27984=CARTESIAN_POINT ( 'NONE',  ( -2.931009552726339784, -14.22630671667915969, 1.500000000000000000 ) ) ;
#27994=PLANE ( 'NONE',  #30208 ) ;
#28005=AXIS2_PLACEMENT_3D ( 'NONE', #27972, #18612, #7053 ) ;
#28015=DIRECTION ( 'NONE',  ( 1.000000000000000000, 0.000000000000000000, 0.000000000000000000 ) ) ;
#28022=ORIENTED_EDGE ( 'NONE', *, *, #11480, .F. ) ;
#28027=VECTOR ( 'NONE', #3382, 1000.000000000000000 ) ;
#28033=LINE ( 'NONE', #16179, #27566 ) ;
#28035=ADVANCED_FACE ( 'NONE', ( #28728 ), #3954, .F. ) ;
#28037=EDGE_CURVE ( 'NONE', #4581, #27445, #491, .T. ) ;
#28038=LINE ( 'NONE', #6665, #4075 ) ;
#28052=AXIS2_PLACEMENT_3D ( 'NONE', #29878, #6004, #22670 ) ;
#28056=CARTESIAN_POINT ( 'NONE',  ( -23.17581250239728519, 34.50630206824672541, -1.499999999999999778 ) ) ;
#28068=AXIS2_PLACEMENT_3D ( 'NONE', #11243, #23081, #20740 ) ;
#28074=EDGE_CURVE ( 'NONE', #13253, #20986, #21795, .T. ) ;
#28083=ORIENTED_EDGE ( 'NONE', *, *, #18625, .T. ) ;
#28121=CYLINDRICAL_SURFACE ( 'NONE', #10808, 1.447898107987170890 ) ;
#28141=VERTEX_POINT ( 'NONE', #11547 ) ;
#28161=CARTESIAN_POINT ( 'NONE',  ( -14.36006998371493637, -17.26937953831884442, 1.500000000000000000 ) ) ;
#28167=ORIENTED_EDGE ( 'NONE', *, *, #15854, .F. ) ;
#28171=ORIENTED_EDGE ( 'NONE', *, *, #25028, .T. ) ;
#28176=CIRCLE ( 'NONE', #15734, 1.447898107987198646 ) ;
#28181=CARTESIAN_POINT ( 'NONE',  ( -30.75232512042845556, -9.966982604840850968, -1.500000000000000000 ) ) ;
#28183=CIRCLE ( 'NONE', #21693, 14.52510309069105965 ) ;
#28185=CARTESIAN_POINT ( 'NONE',  ( -3.221450758838616757, -1.621276839356792454, 1.500000000000000000 ) ) ;
#28191=ORIENTED_EDGE ( 'NONE', *, *, #5617, .T. ) ;
#28200=DIRECTION ( 'NONE',  ( 1.000000000000000000, 0.000000000000000000, 0.000000000000000000 ) ) ;
#28208=DIRECTION ( 'NONE',  ( 1.000000000000000000, 0.000000000000000000, 0.000000000000000000 ) ) ;
#28248=DIRECTION ( 'NONE',  ( 1.000000000000000000, 0.000000000000000000, 0.000000000000000000 ) ) ;
#28251=DIRECTION ( 'NONE',  ( -0.4495526574063634095, -0.8932538319083086487, 0.000000000000000000 ) ) ;
#28252=ORIENTED_EDGE ( 'NONE', *, *, #12317, .T. ) ;
#28263=FACE_OUTER_BOUND ( 'NONE', #23037, .T. ) ;
#28269=CARTESIAN_POINT ( 'NONE',  ( 28.37932450449293853, 10.51822134874671022, 1.500000000000000000 ) ) ;
#28282=DIRECTION ( 'NONE',  ( 0.000000000000000000, -0.000000000000000000, -1.000000000000000000 ) ) ;
#28289=DIRECTION ( 'NONE',  ( -0.000000000000000000, 0.000000000000000000, 1.000000000000000000 ) ) ;
#28294=ORIENTED_EDGE ( 'NONE', *, *, #2515, .F. ) ;
#28311=AXIS2_PLACEMENT_3D ( 'NONE', #25087, #1542, #3730 ) ;
#28316=CARTESIAN_POINT ( 'NONE',  ( 19.54426622602687758, -37.07991288358297055, -1.499999999999999778 ) ) ;
#28340=VECTOR ( 'NONE', #11631, 1000.000000000000000 ) ;
#28405=CARTESIAN_POINT ( 'NONE',  ( -14.89473990422384198, 17.79239818699320708, 1.500000000000000000 ) ) ;
#28416=EDGE_CURVE ( 'NONE', #4932, #24522, #23303, .T. ) ;
#28417=DIRECTION ( 'NONE',  ( -0.000000000000000000, -0.000000000000000000, -1.000000000000000000 ) ) ;
#28418=DIRECTION ( 'NONE',  ( -0.000000000000000000, -0.000000000000000000, -1.000000000000000000 ) ) ;
#28422=DIRECTION ( 'NONE',  ( -0.000000000000000000, 0.000000000000000000, 1.000000000000000000 ) ) ;
#28435=VERTEX_POINT ( 'NONE', #11279 ) ;
#28439=CARTESIAN_POINT ( 'NONE',  ( 1.073881485057738949, 0.9711784013061123266, 1.500000000000000000 ) ) ;
#28447=EDGE_LOOP ( 'NONE', ( #5265, #10770, #30647, #30845 ) ) ;
#28460=EDGE_LOOP ( 'NONE', ( #3443, #28597, #5197, #17495, #1571, #6639 ) ) ;
#28469=DIRECTION ( 'NONE',  ( 1.000000000000000000, 0.000000000000000000, 0.000000000000000000 ) ) ;
#28479=CARTESIAN_POINT ( 'NONE',  ( 28.79137815760242702, -9.331429872129930914, -1.500000000000000000 ) ) ;
#28487=ORIENTED_EDGE ( 'NONE', *, *, #27489, .T. ) ;
#28491=VECTOR ( 'NONE', #29103, 1000.000000000000000 ) ;
#28495=DIRECTION ( 'NONE',  ( 0.000000000000000000, -0.000000000000000000, -1.000000000000000000 ) ) ;
#28500=LINE ( 'NONE', #21308, #16280 ) ;
#28504=CARTESIAN_POINT ( 'NONE',  ( 43.34097750826427387, 11.89502811014146033, -1.500000000000000000 ) ) ;
#28514=DIRECTION ( 'NONE',  ( 0.000000000000000000, 0.000000000000000000, 1.000000000000000000 ) ) ;
#28518=AXIS2_PLACEMENT_3D ( 'NONE', #4611, #28783, #14436 ) ;
#28535=FACE_BOUND ( 'NONE', #8576, .T. ) ;
#28552=ORIENTED_EDGE ( 'NONE', *, *, #5034, .T. ) ;
#28590=DIRECTION ( 'NONE',  ( 1.000000000000000000, 0.000000000000000000, 0.000000000000000000 ) ) ;
#28595=CARTESIAN_POINT ( 'NONE',  ( -43.34097750826426676, 11.89502811014148698, 1.500000000000000444 ) ) ;
#28596=ORIENTED_EDGE ( 'NONE', *, *, #13563, .T. ) ;
#28597=ORIENTED_EDGE ( 'NONE', *, *, #16630, .F. ) ;
#28601=ORIENTED_EDGE ( 'NONE', *, *, #28801, .F. ) ;
#28602=EDGE_LOOP ( 'NONE', ( #2255, #30692, #26126, #7071 ) ) ;
#28623=PLANE ( 'NONE',  #21883 ) ;
#28649=AXIS2_PLACEMENT_3D ( 'NONE', #23906, #20796, #8965 ) ;
#28655=CARTESIAN_POINT ( 'NONE',  ( 43.34097750826426676, -11.89502811014149941, -1.500000000000000000 ) ) ;
#28670=CARTESIAN_POINT ( 'NONE',  ( -4.163336342344337027E-14, -1.387778780781445676E-14, 1.500000000000000000 ) ) ;
#28672=DIRECTION ( 'NONE',  ( -0.000000000000000000, -0.000000000000000000, -1.000000000000000000 ) ) ;
#28677=CARTESIAN_POINT ( 'NONE',  ( 25.10445388623454477, -25.60065097860747585, 1.500000000000000000 ) ) ;
#28682=ORIENTED_EDGE ( 'NONE', *, *, #1036, .T. ) ;
#28686=CARTESIAN_POINT ( 'NONE',  ( -26.36764545593177900, 31.31467416275353344, -1.500000000000000000 ) ) ;
#28690=FACE_BOUND ( 'NONE', #3820, .T. ) ;
#28728=FACE_OUTER_BOUND ( 'NONE', #28447, .T. ) ;
#28739=AXIS2_PLACEMENT_3D ( 'NONE', #5411, #19742, #1037 ) ;
#28743=CARTESIAN_POINT ( 'NONE',  ( -4.163336342344337027E-14, -1.387778780781445676E-14, -1.500000000000000000 ) ) ;
#28747=DIRECTION ( 'NONE',  ( -0.000000000000000000, 0.000000000000000000, 1.000000000000000000 ) ) ;
#28766=ORIENTED_EDGE ( 'NONE', *, *, #23604, .T. ) ;
#28777=ORIENTED_EDGE ( 'NONE', *, *, #29642, .T. ) ;
#28779=AXIS2_PLACEMENT_3D ( 'NONE', #9469, #2913, #408 ) ;
#28783=DIRECTION ( 'NONE',  ( -0.000000000000000000, -0.000000000000000000, -1.000000000000000000 ) ) ;
#28792=CARTESIAN_POINT ( 'NONE',  ( 19.54426622602687402, -37.07991288358297055, -1.499999999999999778 ) ) ;
#28795=DIRECTION ( 'NONE',  ( 1.000000000000000000, 0.000000000000000000, 0.000000000000000000 ) ) ;
#28801=EDGE_CURVE ( 'NONE', #25490, #18893, #558, .T. ) ;
#28807=EDGE_CURVE ( 'NONE', #6600, #5146, #7377, .T. ) ;
#28825=CARTESIAN_POINT ( 'NONE',  ( 28.34828976096172681, 29.18752572968383419, 1.500000000000000000 ) ) ;
#28827=DIRECTION ( 'NONE',  ( -0.000000000000000000, 0.000000000000000000, 1.000000000000000000 ) ) ;
#28828=CYLINDRICAL_SURFACE ( 'NONE', #993, 12.66227964008302287 ) ;
#28829=EDGE_LOOP ( 'NONE', ( #27823, #29251, #17540, #486 ) ) ;
#28845=CIRCLE ( 'NONE', #1921, 2.898871837527149609 ) ;
#28847=ADVANCED_FACE ( 'NONE', ( #26623 ), #17096, .F. ) ;
#28862=PRODUCT_DEFINITION_SHAPE ( 'NONE', 'NONE',  #7631 ) ;
#28882=ORIENTED_EDGE ( 'NONE', *, *, #6403, .T. ) ;
#28887=DIRECTION ( 'NONE',  ( 1.000000000000000000, 0.000000000000000000, 0.000000000000000000 ) ) ;
#28890=CARTESIAN_POINT ( 'NONE',  ( 19.54426622602689179, 37.07991288358296345, 1.499999999999999778 ) ) ;
#28894=ORIENTED_EDGE ( 'NONE', *, *, #20284, .F. ) ;
#28910=ORIENTED_EDGE ( 'NONE', *, *, #5949, .T. ) ;
#28935=VERTEX_POINT ( 'NONE', #20198 ) ;
#28936=ORIENTED_EDGE ( 'NONE', *, *, #30198, .T. ) ;
#28942=VERTEX_POINT ( 'NONE', #6018 ) ;
#28951=ORIENTED_EDGE ( 'NONE', *, *, #22693, .F. ) ;
#28953=DIRECTION ( 'NONE',  ( -0.000000000000000000, -0.000000000000000000, -1.000000000000000000 ) ) ;
#28961=DIRECTION ( 'NONE',  ( 1.000000000000000000, 0.000000000000000000, 0.000000000000000000 ) ) ;
#28965=AXIS2_PLACEMENT_3D ( 'NONE', #26311, #9477, #12125 ) ;
#28966=DIRECTION ( 'NONE',  ( -1.000000000000000000, 0.000000000000000000, 0.000000000000000000 ) ) ;
#28971=CARTESIAN_POINT ( 'NONE',  ( 3.637110358602582583, 19.99473753024312117, 1.500000000000000000 ) ) ;
#28985=CIRCLE ( 'NONE', #9063, 0.7441270634456955690 ) ;
#29000=ORIENTED_EDGE ( 'NONE', *, *, #19357, .T. ) ;
#29002=EDGE_CURVE ( 'NONE', #14300, #15112, #22821, .T. ) ;
#29014=EDGE_CURVE ( 'NONE', #23725, #6974, #20951, .T. ) ;
#29024=CIRCLE ( 'NONE', #27483, 11.46182693247429718 ) ;
#29031=DIRECTION ( 'NONE',  ( -0.000000000000000000, -0.000000000000000000, -1.000000000000000000 ) ) ;
#29032=CARTESIAN_POINT ( 'NONE',  ( 11.21147646446735102, -30.29926891764210595, 1.500000000000000000 ) ) ;
#29051=AXIS2_PLACEMENT_3D ( 'NONE', #18160, #6461, #10831 ) ;
#29052=ORIENTED_EDGE ( 'NONE', *, *, #16253, .F. ) ;
#29062=ORIENTED_EDGE ( 'NONE', *, *, #26046, .T. ) ;
#29063=DIRECTION ( 'NONE',  ( -0.7416830501633135952, -0.6707505147970024284, 0.000000000000000000 ) ) ;
#29086=EDGE_LOOP ( 'NONE', ( #20402, #2672, #11148, #1276 ) ) ;
#29087=CYLINDRICAL_SURFACE ( 'NONE', #20006, 23.20393738267408779 ) ;
#29102=CARTESIAN_POINT ( 'NONE',  ( -9.301547456646385825, 8.591538895647085283, -1.500000000000000000 ) ) ;
#29103=DIRECTION ( 'NONE',  ( -0.000000000000000000, -0.000000000000000000, -1.000000000000000000 ) ) ;
#29106=ORIENTED_EDGE ( 'NONE', *, *, #9757, .F. ) ;
#29108=CARTESIAN_POINT ( 'NONE',  ( 3.118309183252346628, 17.14266753270391774, -1.500000000000000000 ) ) ;
#29126=CARTESIAN_POINT ( 'NONE',  ( 8.616279238414451314, -7.781333699927420966, -1.500000000000000000 ) ) ;
#29131=ORIENTED_EDGE ( 'NONE', *, *, #20617, .F. ) ;
#29137=EDGE_LOOP ( 'NONE', ( #7733, #5378, #8549, #9526 ) ) ;
#29140=ORIENTED_EDGE ( 'NONE', *, *, #3490, .T. ) ;
#29147=DIRECTION ( 'NONE',  ( 0.000000000000000000, -0.000000000000000000, -1.000000000000000000 ) ) ;
#29149=ORIENTED_EDGE ( 'NONE', *, *, #28074, .T. ) ;
#29163=FACE_OUTER_BOUND ( 'NONE', #6006, .T. ) ;
#29180=DIRECTION ( 'NONE',  ( -0.000000000000000000, -0.000000000000000000, -1.000000000000000000 ) ) ;
#29182=CARTESIAN_POINT ( 'NONE',  ( -24.03057240117691862, 26.57182937991349903, 1.500000000000000000 ) ) ;
#29209=ORIENTED_EDGE ( 'NONE', *, *, #17583, .F. ) ;
#29215=DIRECTION ( 'NONE',  ( -0.000000000000000000, 0.000000000000000000, 1.000000000000000000 ) ) ;
#29220=DIRECTION ( 'NONE',  ( -0.000000000000000000, 0.000000000000000000, 1.000000000000000000 ) ) ;
#29222=CARTESIAN_POINT ( 'NONE',  ( -4.100931858250869588, 19.90478481566557178, -1.500000000000000000 ) ) ;
#29232=CARTESIAN_POINT ( 'NONE',  ( -17.22181377296915272, -14.41708049311147555, 1.500000000000000000 ) ) ;
#29244=ORIENTED_EDGE ( 'NONE', *, *, #4768, .F. ) ;
#29251=ORIENTED_EDGE ( 'NONE', *, *, #9991, .T. ) ;
#29262=VECTOR ( 'NONE', #11727, 1000.000000000000000 ) ;
#29265=CIRCLE ( 'NONE', #13331, 28.20443790117963800 ) ;
#29270=DIRECTION ( 'NONE',  ( -0.000000000000000000, -0.000000000000000000, -1.000000000000000000 ) ) ;
#29280=CARTESIAN_POINT ( 'NONE',  ( -9.675133109038686285, -8.168544852422948921, -1.500000000000000000 ) ) ;
#29293=AXIS2_PLACEMENT_3D ( 'NONE', #706, #10537, #1329 ) ;
#29294=CARTESIAN_POINT ( 'NONE',  ( -30.75232512042845556, -9.966982604840850968, 1.500000000000000000 ) ) ;
#29296=AXIS2_PLACEMENT_3D ( 'NONE', #6279, #15636, #3794 ) ;
#29311=CARTESIAN_POINT ( 'NONE',  ( -28.34828976096172681, 29.18752572968383419, -1.500000000000000000 ) ) ;
#29316=CIRCLE ( 'NONE', #10883, 21.71568325578132530 ) ;
#29353=DIRECTION ( 'NONE',  ( 1.000000000000000000, 0.000000000000000000, 0.000000000000000000 ) ) ;
#29381=VECTOR ( 'NONE', #1782, 1000.000000000000000 ) ;
#29395=CARTESIAN_POINT ( 'NONE',  ( -3.515970705488605130, 17.06554576617236307, 1.500000000000000000 ) ) ;
#29399=ORIENTED_EDGE ( 'NONE', *, *, #21972, .F. ) ;
#29408=AXIS2_PLACEMENT_3D ( 'NONE', #8011, #24674, #14044 ) ;
#29418=ORIENTED_EDGE ( 'NONE', *, *, #19819, .F. ) ;
#29425=LINE ( 'NONE', #27229, #1862 ) ;
#29440=CARTESIAN_POINT ( 'NONE',  ( 1.073881485057758711, -0.9711784013061475207, 1.500000000000000000 ) ) ;
#29451=AXIS2_PLACEMENT_3D ( 'NONE', #19779, #29147, #29466 ) ;
#29453=( BOUNDED_CURVE ( )  B_SPLINE_CURVE ( 3, ( #5866, #13197, #13050, #3369 ),
 .UNSPECIFIED., .F., .T. ) 
 B_SPLINE_CURVE_WITH_KNOTS ( ( 4, 4 ),
 ( 5.540737561276206868, 5.872433067142492469 ),
 .UNSPECIFIED. ) 
 CURVE ( )  GEOMETRIC_REPRESENTATION_ITEM ( )  RATIONAL_B_SPLINE_CURVE ( ( 1.000000000000000000, 0.9908525036704132205, 0.9908525036704132205, 1.000000000000000000 ) ) 
 REPRESENTATION_ITEM ( '' )  );
#29464=DIRECTION ( 'NONE',  ( -1.000000000000000000, 0.000000000000000000, 0.000000000000000000 ) ) ;
#29466=DIRECTION ( 'NONE',  ( 1.000000000000000000, 0.000000000000000000, 0.000000000000000000 ) ) ;
#29475=ORIENTED_EDGE ( 'NONE', *, *, #16409, .F. ) ;
#29482=DIRECTION ( 'NONE',  ( -0.000000000000000000, 0.000000000000000000, 1.000000000000000000 ) ) ;
#29483=DIRECTION ( 'NONE',  ( -0.000000000000000000, -0.000000000000000000, -1.000000000000000000 ) ) ;
#29490=CARTESIAN_POINT ( 'NONE',  ( -16.65122935894506639, -13.93942108199812324, 1.500000000000000000 ) ) ;
#29538=EDGE_LOOP ( 'NONE', ( #18129, #16956, #22479, #12810 ) ) ;
#29542=VECTOR ( 'NONE', #21894, 1000.000000000000000 ) ;
#29550=VERTEX_POINT ( 'NONE', #2993 ) ;
#29551=DIRECTION ( 'NONE',  ( 0.000000000000000000, -0.000000000000000000, -1.000000000000000000 ) ) ;
#29554=LINE ( 'NONE', #26604, #1633 ) ;
#29557=DIRECTION ( 'NONE',  ( 0.000000000000000000, -0.000000000000000000, -1.000000000000000000 ) ) ;
#29558=ADVANCED_FACE ( 'NONE', ( #5788 ), #12666, .F. ) ;
#29562=CIRCLE ( 'NONE', #7159, 1.447898107987170890 ) ;
#29563=CARTESIAN_POINT ( 'NONE',  ( 8.260402557893151254, 8.184276679720483116, 1.500000000000000000 ) ) ;
#29575=EDGE_CURVE ( 'NONE', #20986, #10442, #7989, .T. ) ;
#29594=EDGE_CURVE ( 'NONE', #17335, #8993, #3452, .T. ) ;
#29597=ORIENTED_EDGE ( 'NONE', *, *, #9045, .T. ) ;
#29605=CARTESIAN_POINT ( 'NONE',  ( 28.34828976096172681, -29.18752572968383419, 1.500000000000000000 ) ) ;
#29618=PLANE ( 'NONE',  #30282 ) ;
#29630=DIRECTION ( 'NONE',  ( -0.000000000000000000, 0.000000000000000000, 1.000000000000000000 ) ) ;
#29633=AXIS2_PLACEMENT_3D ( 'NONE', #12533, #2697, #19848 ) ;
#29636=CARTESIAN_POINT ( 'NONE',  ( 26.44644203219471379, 9.801837641955973623, 1.500000000000000000 ) ) ;
#29640=CARTESIAN_POINT ( 'NONE',  ( 16.69721919944051791, -13.88429941593332551, 1.500000000000000000 ) ) ;
#29642=EDGE_CURVE ( 'NONE', #27365, #26376, #16876, .T. ) ;
#29646=ORIENTED_EDGE ( 'NONE', *, *, #15630, .T. ) ;
#29648=FACE_OUTER_BOUND ( 'NONE', #20717, .T. ) ;
#29655=CARTESIAN_POINT ( 'NONE',  ( -4.163336342344337027E-14, -1.387778780781445676E-14, 1.500000000000000000 ) ) ;
#29665=DIRECTION ( 'NONE',  ( -0.000000000000000000, -0.000000000000000000, -1.000000000000000000 ) ) ;
#29670=EDGE_LOOP ( 'NONE', ( #25505, #23375, #9200, #7637 ) ) ;
#29671=DIRECTION ( 'NONE',  ( -1.000000000000000000, 0.000000000000000000, 0.000000000000000000 ) ) ;
#29687=CARTESIAN_POINT ( 'NONE',  ( 19.54426622602687402, -37.07991288358297055, 1.499999999999999778 ) ) ;
#29691=FACE_OUTER_BOUND ( 'NONE', #16399, .T. ) ;
#29705=ORIENTED_EDGE ( 'NONE', *, *, #14737, .T. ) ;
#29725=DIRECTION ( 'NONE',  ( 1.000000000000000000, 0.000000000000000000, 0.000000000000000000 ) ) ;
#29730=CARTESIAN_POINT ( 'NONE',  ( 16.52525247487311333, -14.36006998371588317, 1.500000000000000000 ) ) ;
#29744=DIRECTION ( 'NONE',  ( -0.000000000000000000, 0.000000000000000000, 1.000000000000000000 ) ) ;
#29750=AXIS2_PLACEMENT_3D ( 'NONE', #22240, #14919, #22081 ) ;
#29776=VERTEX_POINT ( 'NONE', #14574 ) ;
#29785=CARTESIAN_POINT ( 'NONE',  ( -4.163336342344337027E-14, -1.387778780781445676E-14, 1.500000000000000000 ) ) ;
#29824=CARTESIAN_POINT ( 'NONE',  ( -28.37932450449293853, 10.51822134874671022, -1.500000000000000000 ) ) ;
#29835=CARTESIAN_POINT ( 'NONE',  ( 0.000000000000000000, 0.000000000000000000, -1.500000000000000000 ) ) ;
#29844=DIRECTION ( 'NONE',  ( -1.000000000000000000, 0.000000000000000000, 0.000000000000000000 ) ) ;
#29846=ORIENTED_EDGE ( 'NONE', *, *, #1036, .F. ) ;
#29847=CARTESIAN_POINT ( 'NONE',  ( 0.000000000000000000, 0.000000000000000000, 1.500000000000000000 ) ) ;
#29861=ORIENTED_EDGE ( 'NONE', *, *, #30016, .T. ) ;
#29862=CIRCLE ( 'NONE', #3469, 0.7441270634457181066 ) ;
#29864=CARTESIAN_POINT ( 'NONE',  ( -26.36764545593177544, 31.31467416275353344, -1.500000000000000000 ) ) ;
#29873=CARTESIAN_POINT ( 'NONE',  ( 17.26937953831880534, -14.36006998371588317, 1.500000000000000000 ) ) ;
#29878=CARTESIAN_POINT ( 'NONE',  ( -4.163336342344337027E-14, -1.387778780781445676E-14, 1.500000000000000000 ) ) ;
#29889=DIRECTION ( 'NONE',  ( -0.000000000000000000, -0.000000000000000000, -1.000000000000000000 ) ) ;
#29890=ORIENTED_EDGE ( 'NONE', *, *, #30, .F. ) ;
#29894=DIRECTION ( 'NONE',  ( 0.000000000000000000, -0.000000000000000000, -1.000000000000000000 ) ) ;
#29919=FACE_OUTER_BOUND ( 'NONE', #22248, .T. ) ;
#29935=DIRECTION ( 'NONE',  ( 1.000000000000000000, 0.000000000000000000, 0.000000000000000000 ) ) ;
#29962=CARTESIAN_POINT ( 'NONE',  ( 0.000000000000000000, 0.000000000000000000, 1.500000000000000000 ) ) ;
#29973=DIRECTION ( 'NONE',  ( -0.000000000000000000, -0.000000000000000000, -1.000000000000000000 ) ) ;
#29974=DIRECTION ( 'NONE',  ( -0.000000000000000000, -0.000000000000000000, -1.000000000000000000 ) ) ;
#29983=EDGE_LOOP ( 'NONE', ( #24990, #13471, #21124, #12026, #15, #29149 ) ) ;
#29986=DIRECTION ( 'NONE',  ( 1.000000000000000000, 0.000000000000000000, 0.000000000000000000 ) ) ;
#29992=CARTESIAN_POINT ( 'NONE',  ( 13.88429941593329531, 16.69721919943964039, 1.500000000000000000 ) ) ;
#29993=EDGE_LOOP ( 'NONE', ( #13657, #13677, #10727, #848 ) ) ;
#29999=FACE_OUTER_BOUND ( 'NONE', #7544, .T. ) ;
#30011=CARTESIAN_POINT ( 'NONE',  ( -26.36764545593177544, 31.31467416275353344, 1.500000000000000000 ) ) ;
#30016=EDGE_CURVE ( 'NONE', #22720, #29776, #12889, .T. ) ;
#30017=CARTESIAN_POINT ( 'NONE',  ( 9.301547456646380496, 8.591538895647095941, 1.500000000000000000 ) ) ;
#30031=VERTEX_POINT ( 'NONE', #24258 ) ;
#30061=DIRECTION ( 'NONE',  ( 0.7416830501633135952, 0.6707505147970024284, -0.000000000000000000 ) ) ;
#30067=EDGE_CURVE ( 'NONE', #8808, #25145, #6945, .T. ) ;
#30077=FACE_BOUND ( 'NONE', #28460, .T. ) ;
#30082=ORIENTED_EDGE ( 'NONE', *, *, #16806, .T. ) ;
#30119=LINE ( 'NONE', #27481, #8155 ) ;
#30142=CARTESIAN_POINT ( 'NONE',  ( -4.163336342344337027E-14, -1.387778780781445676E-14, 1.500000000000000000 ) ) ;
#30181=VECTOR ( 'NONE', #2377, 1000.000000000000000 ) ;
#30182=DIRECTION ( 'NONE',  ( -0.000000000000000000, -0.000000000000000000, -1.000000000000000000 ) ) ;
#30198=EDGE_CURVE ( 'NONE', #14669, #584, #22987, .T. ) ;
#30208=AXIS2_PLACEMENT_3D ( 'NONE', #25656, #4275, #11008 ) ;
#30226=LINE ( 'NONE', #6374, #10029 ) ;
#30235=DIRECTION ( 'NONE',  ( -0.000000000000000000, 0.000000000000000000, 1.000000000000000000 ) ) ;
#30244=DIRECTION ( 'NONE',  ( -0.000000000000000000, -0.000000000000000000, -1.000000000000000000 ) ) ;
#30261=VERTEX_POINT ( 'NONE', #24885 ) ;
#30262=CIRCLE ( 'NONE', #16815, 0.7441270634457181066 ) ;
#30272=DIRECTION ( 'NONE',  ( -1.000000000000000000, 0.000000000000000000, 0.000000000000000000 ) ) ;
#30274=( NAMED_UNIT ( * ) PLANE_ANGLE_UNIT ( ) SI_UNIT ( $, .RADIAN. ) );
#30282=AXIS2_PLACEMENT_3D ( 'NONE', #23036, #22894, #8570 ) ;
#30283=FACE_OUTER_BOUND ( 'NONE', #8450, .T. ) ;
#30300=EDGE_LOOP ( 'NONE', ( #21971, #14437, #10938, #6896 ) ) ;
#30302=CIRCLE ( 'NONE', #21319, 0.7441270634456903510 ) ;
#30304=CARTESIAN_POINT ( 'NONE',  ( 24.03057240117691862, -26.57182937991349903, 1.500000000000000000 ) ) ;
#30322=VERTEX_POINT ( 'NONE', #20502 ) ;
#30326=VECTOR ( 'NONE', #12683, 1000.000000000000000 ) ;
#30350=AXIS2_PLACEMENT_3D ( 'NONE', #7412, #24824, #10629 ) ;
#30355=DIRECTION ( 'NONE',  ( 0.000000000000000000, -0.000000000000000000, -1.000000000000000000 ) ) ;
#30359=CIRCLE ( 'NONE', #24884, 0.6002263538043630664 ) ;
#30375=CARTESIAN_POINT ( 'NONE',  ( 2.599508007902112006, -14.29059753516471964, 1.500000000000000000 ) ) ;
#30379=CYLINDRICAL_SURFACE ( 'NONE', #1346, 0.7441270634456903510 ) ;
#30383=DIRECTION ( 'NONE',  ( -0.000000000000000000, -0.000000000000000000, -1.000000000000000000 ) ) ;
#30387=EDGE_LOOP ( 'NONE', ( #28171, #3718, #4880, #8386 ) ) ;
#30388=EDGE_CURVE ( 'NONE', #24914, #14826, #17344, .T. ) ;
#30389=ADVANCED_FACE ( 'NONE', ( #800 ), #22331, .F. ) ;
#30394=ORIENTED_EDGE ( 'NONE', *, *, #11301, .T. ) ;
#30405=CARTESIAN_POINT ( 'NONE',  ( 13.93942108199810193, -16.65122935894600076, 1.500000000000000000 ) ) ;
#30409=EDGE_LOOP ( 'NONE', ( #27925, #14229, #22712, #29062 ) ) ;
#30447=DIRECTION ( 'NONE',  ( 1.000000000000000000, 0.000000000000000000, 0.000000000000000000 ) ) ;
#30478=CARTESIAN_POINT ( 'NONE',  ( -4.163336342344337027E-14, 1.387778780781445676E-14, 1.500000000000000000 ) ) ;
#30485=DIRECTION ( 'NONE',  ( -0.000000000000000000, -0.000000000000000000, -1.000000000000000000 ) ) ;
#30520=FACE_OUTER_BOUND ( 'NONE', #29137, .T. ) ;
#30522=CARTESIAN_POINT ( 'NONE',  ( 28.34828976096172681, -29.18752572968383419, -1.500000000000000000 ) ) ;
#30536=VECTOR ( 'NONE', #19567, 1000.000000000000000 ) ;
#30542=CARTESIAN_POINT ( 'NONE',  ( -26.36764545593177544, 31.31467416275353344, -1.500000000000000000 ) ) ;
#30547=ORIENTED_EDGE ( 'NONE', *, *, #16891, .F. ) ;
#30548=DIRECTION ( 'NONE',  ( -1.000000000000000000, 0.000000000000000000, 0.000000000000000000 ) ) ;
#30560=ORIENTED_EDGE ( 'NONE', *, *, #11661, .F. ) ;
#30576=EDGE_LOOP ( 'NONE', ( #4380, #23198, #14068, #19091 ) ) ;
#30587=ORIENTED_EDGE ( 'NONE', *, *, #12250, .T. ) ;
#30633=AXIS2_PLACEMENT_3D ( 'NONE', #9522, #16092, #4228 ) ;
#30634=LINE ( 'NONE', #20961, #16015 ) ;
#30637=LINE ( 'NONE', #4750, #21532 ) ;
#30647=ORIENTED_EDGE ( 'NONE', *, *, #9922, .F. ) ;
#30690=ORIENTED_EDGE ( 'NONE', *, *, #26381, .T. ) ;
#30692=ORIENTED_EDGE ( 'NONE', *, *, #9738, .F. ) ;
#30696=EDGE_CURVE ( 'NONE', #19427, #12321, #10280, .T. ) ;
#30703=DIRECTION ( 'NONE',  ( 1.000000000000000000, 0.000000000000000000, 0.000000000000000000 ) ) ;
#30723=AXIS2_PLACEMENT_3D ( 'NONE', #14453, #23956, #16486 ) ;
#30745=CARTESIAN_POINT ( 'NONE',  ( 14.36006998371584054, 17.26937953831785677, -1.500000000000000000 ) ) ;
#30753=CARTESIAN_POINT ( 'NONE',  ( 23.17581250239729940, 34.50630206824671120, 1.499999999999999778 ) ) ;
#30756=DIRECTION ( 'NONE',  ( 0.000000000000000000, -0.000000000000000000, -1.000000000000000000 ) ) ;
#30777=VERTEX_POINT ( 'NONE', #2467 ) ;
#30821=DIRECTION ( 'NONE',  ( -0.000000000000000000, -0.000000000000000000, -1.000000000000000000 ) ) ;
#30823=FACE_OUTER_BOUND ( 'NONE', #5072, .T. ) ;
#30834=ORIENTED_EDGE ( 'NONE', *, *, #26547, .F. ) ;
#30844=CARTESIAN_POINT ( 'NONE',  ( -4.163336342344337027E-14, -1.387778780781445676E-14, 1.500000000000000000 ) ) ;
#30845=ORIENTED_EDGE ( 'NONE', *, *, #23433, .T. ) ;
#30850=CYLINDRICAL_SURFACE ( 'NONE', #20766, 21.71568325578202163 ) ;
#30880=COLOUR_RGB('Light Blue',0.38,0.62,0.78);
#30881=FILL_AREA_STYLE_COLOUR('',#30880);
#30882=FILL_AREA_STYLE('',(#30881));
#30883=SURFACE_STYLE_FILL_AREA(#30882);
#30884=SURFACE_SIDE_STYLE('',(#30883));
#30885=SURFACE_STYLE_USAGE(.BOTH.,#30884);
#30886=PRESENTATION_STYLE_ASSIGNMENT((#30885));
ENDSEC;
END-ISO-10303-21;
